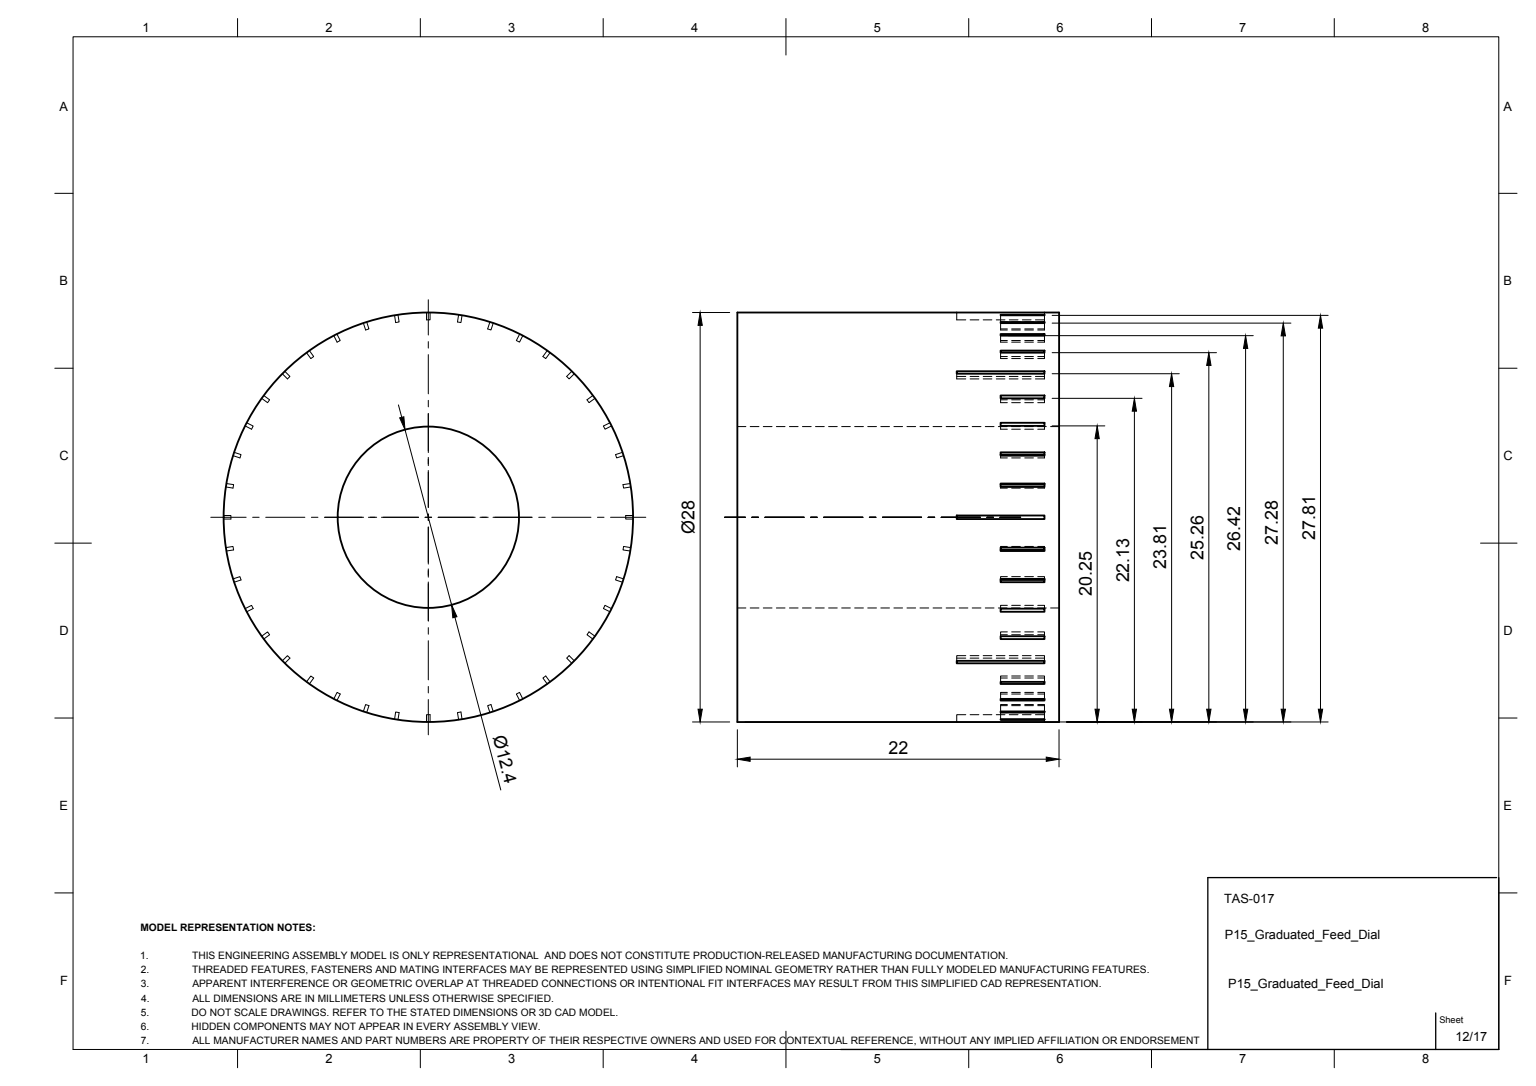
ISO-10303-21;
HEADER;
/* Generated by software containing ST-Developer
 * from STEP Tools, Inc. (www.steptools.com) 
 */

FILE_DESCRIPTION(
/* description */ ('STEP AP203'),
/* implementation_level */ '2;1');

FILE_NAME(
/* name */ 'P15_Graduated_Feed_Dial.step',
/* time_stamp */ '2026-11-15T15:04:01-08:00',
/* author */ (''),
/* organization */ (''),
/* preprocessor_version */ 'ST-DEVELOPER v20.2',
/* originating_system */ 'Autodesk Translation Framework v15.17.0.0',
/* authorisation */ '');

FILE_SCHEMA (('AUTOMOTIVE_DESIGN { 1 0 10303 214 3 1 1 }'));
ENDSEC;

DATA;
#10=MECHANICAL_DESIGN_GEOMETRIC_PRESENTATION_REPRESENTATION('',(#298),#16598);
#220=SHAPE_REPRESENTATION_RELATIONSHIP('SRR','None',#16714,#244);
#244=ADVANCED_BREP_SHAPE_REPRESENTATION('',(#268),#16590);
#268=MANIFOLD_SOLID_BREP('Body1',#9803);
#298=STYLED_ITEM('',(#16834),#268);
#374=FACE_BOUND('',#1807,.T.);
#375=FACE_BOUND('',#1808,.T.);
#376=FACE_BOUND('',#1809,.T.);
#377=FACE_BOUND('',#1810,.T.);
#378=FACE_BOUND('',#1811,.T.);
#379=FACE_BOUND('',#1812,.T.);
#380=FACE_BOUND('',#1813,.T.);
#381=FACE_BOUND('',#1814,.T.);
#382=FACE_BOUND('',#1815,.T.);
#383=FACE_BOUND('',#1816,.T.);
#384=FACE_BOUND('',#1817,.T.);
#385=FACE_BOUND('',#1818,.T.);
#386=FACE_BOUND('',#1819,.T.);
#387=FACE_BOUND('',#1820,.T.);
#388=FACE_BOUND('',#1821,.T.);
#389=FACE_BOUND('',#1822,.T.);
#390=FACE_BOUND('',#1823,.T.);
#391=FACE_BOUND('',#1824,.T.);
#392=FACE_BOUND('',#1825,.T.);
#393=FACE_BOUND('',#1826,.T.);
#394=FACE_BOUND('',#1827,.T.);
#395=FACE_BOUND('',#1828,.T.);
#396=FACE_BOUND('',#1829,.T.);
#397=FACE_BOUND('',#1830,.T.);
#398=FACE_BOUND('',#1831,.T.);
#399=FACE_BOUND('',#1832,.T.);
#400=FACE_BOUND('',#1833,.T.);
#401=FACE_BOUND('',#1834,.T.);
#402=FACE_BOUND('',#1835,.T.);
#403=FACE_BOUND('',#1836,.T.);
#404=FACE_BOUND('',#1837,.T.);
#405=FACE_BOUND('',#1838,.T.);
#406=FACE_BOUND('',#1839,.T.);
#407=FACE_BOUND('',#1840,.T.);
#408=FACE_BOUND('',#1841,.T.);
#409=FACE_BOUND('',#1842,.T.);
#410=FACE_BOUND('',#1843,.T.);
#411=FACE_BOUND('',#1844,.T.);
#412=FACE_BOUND('',#1845,.T.);
#413=FACE_BOUND('',#1847,.T.);
#414=FACE_BOUND('',#1849,.T.);
#651=PLANE('',#10576);
#652=PLANE('',#10577);
#653=PLANE('',#10578);
#654=PLANE('',#10579);
#655=PLANE('',#10580);
#656=PLANE('',#10581);
#657=PLANE('',#10582);
#658=PLANE('',#10583);
#659=PLANE('',#10584);
#660=PLANE('',#10585);
#661=PLANE('',#10586);
#662=PLANE('',#10587);
#663=PLANE('',#10588);
#664=PLANE('',#10589);
#665=PLANE('',#10590);
#666=PLANE('',#10591);
#667=PLANE('',#10592);
#668=PLANE('',#10593);
#669=PLANE('',#10594);
#670=PLANE('',#10595);
#671=PLANE('',#10596);
#672=PLANE('',#10597);
#673=PLANE('',#10598);
#674=PLANE('',#10599);
#675=PLANE('',#10600);
#676=PLANE('',#10601);
#677=PLANE('',#10602);
#678=PLANE('',#10603);
#679=PLANE('',#10604);
#680=PLANE('',#10605);
#681=PLANE('',#10606);
#682=PLANE('',#10607);
#683=PLANE('',#10608);
#684=PLANE('',#10609);
#685=PLANE('',#10610);
#686=PLANE('',#10611);
#687=PLANE('',#10612);
#688=PLANE('',#10613);
#689=PLANE('',#10614);
#690=PLANE('',#10615);
#691=PLANE('',#10616);
#692=PLANE('',#10617);
#693=PLANE('',#10618);
#694=PLANE('',#10619);
#695=PLANE('',#10620);
#696=PLANE('',#10621);
#697=PLANE('',#10622);
#698=PLANE('',#10623);
#699=PLANE('',#10624);
#700=PLANE('',#10625);
#701=PLANE('',#10626);
#702=PLANE('',#10627);
#703=PLANE('',#10628);
#704=PLANE('',#10629);
#705=PLANE('',#10630);
#706=PLANE('',#10631);
#707=PLANE('',#10632);
#708=PLANE('',#10633);
#709=PLANE('',#10634);
#710=PLANE('',#10635);
#711=PLANE('',#10636);
#712=PLANE('',#10637);
#713=PLANE('',#10638);
#714=PLANE('',#10639);
#715=PLANE('',#10640);
#716=PLANE('',#10641);
#717=PLANE('',#10642);
#718=PLANE('',#10643);
#719=PLANE('',#10644);
#720=PLANE('',#10645);
#721=PLANE('',#10646);
#722=PLANE('',#10647);
#723=PLANE('',#10648);
#724=PLANE('',#10649);
#725=PLANE('',#10650);
#726=PLANE('',#10651);
#727=PLANE('',#10652);
#728=PLANE('',#10653);
#729=PLANE('',#10654);
#730=PLANE('',#10655);
#731=PLANE('',#10656);
#732=PLANE('',#10657);
#733=PLANE('',#10658);
#734=PLANE('',#10659);
#735=PLANE('',#10660);
#736=PLANE('',#10661);
#737=PLANE('',#10662);
#738=PLANE('',#10663);
#739=PLANE('',#10664);
#740=PLANE('',#10665);
#741=PLANE('',#10666);
#742=PLANE('',#10667);
#743=PLANE('',#10668);
#744=PLANE('',#10669);
#745=PLANE('',#10670);
#746=PLANE('',#10671);
#747=PLANE('',#10672);
#748=PLANE('',#10673);
#749=PLANE('',#10674);
#750=PLANE('',#10675);
#751=PLANE('',#10676);
#752=PLANE('',#10677);
#753=PLANE('',#10678);
#754=PLANE('',#10679);
#755=PLANE('',#10680);
#756=PLANE('',#10681);
#757=PLANE('',#10682);
#758=PLANE('',#10683);
#759=PLANE('',#10684);
#760=PLANE('',#10685);
#761=PLANE('',#10686);
#762=PLANE('',#10687);
#763=PLANE('',#10688);
#764=PLANE('',#10689);
#765=PLANE('',#10690);
#766=PLANE('',#10691);
#767=PLANE('',#10692);
#768=PLANE('',#10693);
#769=PLANE('',#10694);
#770=PLANE('',#10695);
#771=PLANE('',#10696);
#772=PLANE('',#10697);
#773=PLANE('',#10698);
#774=PLANE('',#10699);
#775=PLANE('',#10700);
#776=PLANE('',#10701);
#777=PLANE('',#10702);
#778=PLANE('',#10703);
#779=PLANE('',#10704);
#780=PLANE('',#10705);
#781=PLANE('',#10706);
#782=PLANE('',#10707);
#783=PLANE('',#10708);
#784=PLANE('',#10709);
#785=PLANE('',#10710);
#786=PLANE('',#10711);
#787=PLANE('',#10712);
#788=PLANE('',#10713);
#789=PLANE('',#10714);
#790=PLANE('',#10715);
#791=PLANE('',#10716);
#792=PLANE('',#10717);
#793=PLANE('',#10718);
#794=PLANE('',#10719);
#795=PLANE('',#10720);
#796=PLANE('',#10721);
#797=PLANE('',#10722);
#798=PLANE('',#10723);
#799=PLANE('',#10724);
#800=PLANE('',#10725);
#801=PLANE('',#10726);
#802=PLANE('',#10727);
#803=PLANE('',#10728);
#804=PLANE('',#10729);
#805=PLANE('',#10730);
#806=PLANE('',#10731);
#807=PLANE('',#10732);
#808=PLANE('',#10733);
#809=PLANE('',#10734);
#810=PLANE('',#10735);
#811=PLANE('',#10736);
#812=PLANE('',#10737);
#813=PLANE('',#10738);
#814=PLANE('',#10739);
#815=PLANE('',#10740);
#816=PLANE('',#10741);
#817=PLANE('',#10742);
#818=PLANE('',#10743);
#819=PLANE('',#10744);
#820=PLANE('',#10745);
#821=PLANE('',#10746);
#822=PLANE('',#10747);
#823=PLANE('',#10748);
#824=PLANE('',#10749);
#825=PLANE('',#10750);
#826=PLANE('',#10751);
#827=PLANE('',#10752);
#828=PLANE('',#10753);
#829=PLANE('',#10754);
#830=PLANE('',#10755);
#831=PLANE('',#10756);
#832=PLANE('',#10757);
#833=PLANE('',#10758);
#834=PLANE('',#10759);
#835=PLANE('',#10760);
#836=PLANE('',#10761);
#837=PLANE('',#10762);
#838=PLANE('',#10763);
#839=PLANE('',#10764);
#840=PLANE('',#10765);
#841=PLANE('',#10766);
#842=PLANE('',#10767);
#843=PLANE('',#10768);
#844=PLANE('',#10769);
#845=PLANE('',#10770);
#846=PLANE('',#10771);
#847=PLANE('',#10772);
#848=PLANE('',#10773);
#849=PLANE('',#10774);
#850=PLANE('',#10775);
#851=PLANE('',#10776);
#852=PLANE('',#10777);
#1186=FACE_OUTER_BOUND('',#1805,.T.);
#1187=FACE_OUTER_BOUND('',#1806,.T.);
#1188=FACE_OUTER_BOUND('',#1846,.T.);
#1189=FACE_OUTER_BOUND('',#1848,.T.);
#1190=FACE_OUTER_BOUND('',#1850,.T.);
#1191=FACE_OUTER_BOUND('',#1851,.T.);
#1192=FACE_OUTER_BOUND('',#1852,.T.);
#1193=FACE_OUTER_BOUND('',#1853,.T.);
#1194=FACE_OUTER_BOUND('',#1854,.T.);
#1195=FACE_OUTER_BOUND('',#1855,.T.);
#1196=FACE_OUTER_BOUND('',#1856,.T.);
#1197=FACE_OUTER_BOUND('',#1857,.T.);
#1198=FACE_OUTER_BOUND('',#1858,.T.);
#1199=FACE_OUTER_BOUND('',#1859,.T.);
#1200=FACE_OUTER_BOUND('',#1860,.T.);
#1201=FACE_OUTER_BOUND('',#1861,.T.);
#1202=FACE_OUTER_BOUND('',#1862,.T.);
#1203=FACE_OUTER_BOUND('',#1863,.T.);
#1204=FACE_OUTER_BOUND('',#1864,.T.);
#1205=FACE_OUTER_BOUND('',#1865,.T.);
#1206=FACE_OUTER_BOUND('',#1866,.T.);
#1207=FACE_OUTER_BOUND('',#1867,.T.);
#1208=FACE_OUTER_BOUND('',#1868,.T.);
#1209=FACE_OUTER_BOUND('',#1869,.T.);
#1210=FACE_OUTER_BOUND('',#1870,.T.);
#1211=FACE_OUTER_BOUND('',#1871,.T.);
#1212=FACE_OUTER_BOUND('',#1872,.T.);
#1213=FACE_OUTER_BOUND('',#1873,.T.);
#1214=FACE_OUTER_BOUND('',#1874,.T.);
#1215=FACE_OUTER_BOUND('',#1875,.T.);
#1216=FACE_OUTER_BOUND('',#1876,.T.);
#1217=FACE_OUTER_BOUND('',#1877,.T.);
#1218=FACE_OUTER_BOUND('',#1878,.T.);
#1219=FACE_OUTER_BOUND('',#1879,.T.);
#1220=FACE_OUTER_BOUND('',#1880,.T.);
#1221=FACE_OUTER_BOUND('',#1881,.T.);
#1222=FACE_OUTER_BOUND('',#1882,.T.);
#1223=FACE_OUTER_BOUND('',#1883,.T.);
#1224=FACE_OUTER_BOUND('',#1884,.T.);
#1225=FACE_OUTER_BOUND('',#1885,.T.);
#1226=FACE_OUTER_BOUND('',#1886,.T.);
#1227=FACE_OUTER_BOUND('',#1887,.T.);
#1228=FACE_OUTER_BOUND('',#1888,.T.);
#1229=FACE_OUTER_BOUND('',#1889,.T.);
#1230=FACE_OUTER_BOUND('',#1890,.T.);
#1231=FACE_OUTER_BOUND('',#1891,.T.);
#1232=FACE_OUTER_BOUND('',#1892,.T.);
#1233=FACE_OUTER_BOUND('',#1893,.T.);
#1234=FACE_OUTER_BOUND('',#1894,.T.);
#1235=FACE_OUTER_BOUND('',#1895,.T.);
#1236=FACE_OUTER_BOUND('',#1896,.T.);
#1237=FACE_OUTER_BOUND('',#1897,.T.);
#1238=FACE_OUTER_BOUND('',#1898,.T.);
#1239=FACE_OUTER_BOUND('',#1899,.T.);
#1240=FACE_OUTER_BOUND('',#1900,.T.);
#1241=FACE_OUTER_BOUND('',#1901,.T.);
#1242=FACE_OUTER_BOUND('',#1902,.T.);
#1243=FACE_OUTER_BOUND('',#1903,.T.);
#1244=FACE_OUTER_BOUND('',#1904,.T.);
#1245=FACE_OUTER_BOUND('',#1905,.T.);
#1246=FACE_OUTER_BOUND('',#1906,.T.);
#1247=FACE_OUTER_BOUND('',#1907,.T.);
#1248=FACE_OUTER_BOUND('',#1908,.T.);
#1249=FACE_OUTER_BOUND('',#1909,.T.);
#1250=FACE_OUTER_BOUND('',#1910,.T.);
#1251=FACE_OUTER_BOUND('',#1911,.T.);
#1252=FACE_OUTER_BOUND('',#1912,.T.);
#1253=FACE_OUTER_BOUND('',#1913,.T.);
#1254=FACE_OUTER_BOUND('',#1914,.T.);
#1255=FACE_OUTER_BOUND('',#1915,.T.);
#1256=FACE_OUTER_BOUND('',#1916,.T.);
#1257=FACE_OUTER_BOUND('',#1917,.T.);
#1258=FACE_OUTER_BOUND('',#1918,.T.);
#1259=FACE_OUTER_BOUND('',#1919,.T.);
#1260=FACE_OUTER_BOUND('',#1920,.T.);
#1261=FACE_OUTER_BOUND('',#1921,.T.);
#1262=FACE_OUTER_BOUND('',#1922,.T.);
#1263=FACE_OUTER_BOUND('',#1923,.T.);
#1264=FACE_OUTER_BOUND('',#1924,.T.);
#1265=FACE_OUTER_BOUND('',#1925,.T.);
#1266=FACE_OUTER_BOUND('',#1926,.T.);
#1267=FACE_OUTER_BOUND('',#1927,.T.);
#1268=FACE_OUTER_BOUND('',#1928,.T.);
#1269=FACE_OUTER_BOUND('',#1929,.T.);
#1270=FACE_OUTER_BOUND('',#1930,.T.);
#1271=FACE_OUTER_BOUND('',#1931,.T.);
#1272=FACE_OUTER_BOUND('',#1932,.T.);
#1273=FACE_OUTER_BOUND('',#1933,.T.);
#1274=FACE_OUTER_BOUND('',#1934,.T.);
#1275=FACE_OUTER_BOUND('',#1935,.T.);
#1276=FACE_OUTER_BOUND('',#1936,.T.);
#1277=FACE_OUTER_BOUND('',#1937,.T.);
#1278=FACE_OUTER_BOUND('',#1938,.T.);
#1279=FACE_OUTER_BOUND('',#1939,.T.);
#1280=FACE_OUTER_BOUND('',#1940,.T.);
#1281=FACE_OUTER_BOUND('',#1941,.T.);
#1282=FACE_OUTER_BOUND('',#1942,.T.);
#1283=FACE_OUTER_BOUND('',#1943,.T.);
#1284=FACE_OUTER_BOUND('',#1944,.T.);
#1285=FACE_OUTER_BOUND('',#1945,.T.);
#1286=FACE_OUTER_BOUND('',#1946,.T.);
#1287=FACE_OUTER_BOUND('',#1947,.T.);
#1288=FACE_OUTER_BOUND('',#1948,.T.);
#1289=FACE_OUTER_BOUND('',#1949,.T.);
#1290=FACE_OUTER_BOUND('',#1950,.T.);
#1291=FACE_OUTER_BOUND('',#1951,.T.);
#1292=FACE_OUTER_BOUND('',#1952,.T.);
#1293=FACE_OUTER_BOUND('',#1953,.T.);
#1294=FACE_OUTER_BOUND('',#1954,.T.);
#1295=FACE_OUTER_BOUND('',#1955,.T.);
#1296=FACE_OUTER_BOUND('',#1956,.T.);
#1297=FACE_OUTER_BOUND('',#1957,.T.);
#1298=FACE_OUTER_BOUND('',#1958,.T.);
#1299=FACE_OUTER_BOUND('',#1959,.T.);
#1300=FACE_OUTER_BOUND('',#1960,.T.);
#1301=FACE_OUTER_BOUND('',#1961,.T.);
#1302=FACE_OUTER_BOUND('',#1962,.T.);
#1303=FACE_OUTER_BOUND('',#1963,.T.);
#1304=FACE_OUTER_BOUND('',#1964,.T.);
#1305=FACE_OUTER_BOUND('',#1965,.T.);
#1306=FACE_OUTER_BOUND('',#1966,.T.);
#1307=FACE_OUTER_BOUND('',#1967,.T.);
#1308=FACE_OUTER_BOUND('',#1968,.T.);
#1309=FACE_OUTER_BOUND('',#1969,.T.);
#1310=FACE_OUTER_BOUND('',#1970,.T.);
#1311=FACE_OUTER_BOUND('',#1971,.T.);
#1312=FACE_OUTER_BOUND('',#1972,.T.);
#1313=FACE_OUTER_BOUND('',#1973,.T.);
#1314=FACE_OUTER_BOUND('',#1974,.T.);
#1315=FACE_OUTER_BOUND('',#1975,.T.);
#1316=FACE_OUTER_BOUND('',#1976,.T.);
#1317=FACE_OUTER_BOUND('',#1977,.T.);
#1318=FACE_OUTER_BOUND('',#1978,.T.);
#1319=FACE_OUTER_BOUND('',#1979,.T.);
#1320=FACE_OUTER_BOUND('',#1980,.T.);
#1321=FACE_OUTER_BOUND('',#1981,.T.);
#1322=FACE_OUTER_BOUND('',#1982,.T.);
#1323=FACE_OUTER_BOUND('',#1983,.T.);
#1324=FACE_OUTER_BOUND('',#1984,.T.);
#1325=FACE_OUTER_BOUND('',#1985,.T.);
#1326=FACE_OUTER_BOUND('',#1986,.T.);
#1327=FACE_OUTER_BOUND('',#1987,.T.);
#1328=FACE_OUTER_BOUND('',#1988,.T.);
#1329=FACE_OUTER_BOUND('',#1989,.T.);
#1330=FACE_OUTER_BOUND('',#1990,.T.);
#1331=FACE_OUTER_BOUND('',#1991,.T.);
#1332=FACE_OUTER_BOUND('',#1992,.T.);
#1333=FACE_OUTER_BOUND('',#1993,.T.);
#1334=FACE_OUTER_BOUND('',#1994,.T.);
#1335=FACE_OUTER_BOUND('',#1995,.T.);
#1336=FACE_OUTER_BOUND('',#1996,.T.);
#1337=FACE_OUTER_BOUND('',#1997,.T.);
#1338=FACE_OUTER_BOUND('',#1998,.T.);
#1339=FACE_OUTER_BOUND('',#1999,.T.);
#1340=FACE_OUTER_BOUND('',#2000,.T.);
#1341=FACE_OUTER_BOUND('',#2001,.T.);
#1342=FACE_OUTER_BOUND('',#2002,.T.);
#1343=FACE_OUTER_BOUND('',#2003,.T.);
#1344=FACE_OUTER_BOUND('',#2004,.T.);
#1345=FACE_OUTER_BOUND('',#2005,.T.);
#1346=FACE_OUTER_BOUND('',#2006,.T.);
#1347=FACE_OUTER_BOUND('',#2007,.T.);
#1348=FACE_OUTER_BOUND('',#2008,.T.);
#1349=FACE_OUTER_BOUND('',#2009,.T.);
#1350=FACE_OUTER_BOUND('',#2010,.T.);
#1351=FACE_OUTER_BOUND('',#2011,.T.);
#1352=FACE_OUTER_BOUND('',#2012,.T.);
#1353=FACE_OUTER_BOUND('',#2013,.T.);
#1354=FACE_OUTER_BOUND('',#2014,.T.);
#1355=FACE_OUTER_BOUND('',#2015,.T.);
#1356=FACE_OUTER_BOUND('',#2016,.T.);
#1357=FACE_OUTER_BOUND('',#2017,.T.);
#1358=FACE_OUTER_BOUND('',#2018,.T.);
#1359=FACE_OUTER_BOUND('',#2019,.T.);
#1360=FACE_OUTER_BOUND('',#2020,.T.);
#1361=FACE_OUTER_BOUND('',#2021,.T.);
#1362=FACE_OUTER_BOUND('',#2022,.T.);
#1363=FACE_OUTER_BOUND('',#2023,.T.);
#1364=FACE_OUTER_BOUND('',#2024,.T.);
#1365=FACE_OUTER_BOUND('',#2025,.T.);
#1366=FACE_OUTER_BOUND('',#2026,.T.);
#1367=FACE_OUTER_BOUND('',#2027,.T.);
#1368=FACE_OUTER_BOUND('',#2028,.T.);
#1369=FACE_OUTER_BOUND('',#2029,.T.);
#1370=FACE_OUTER_BOUND('',#2030,.T.);
#1371=FACE_OUTER_BOUND('',#2031,.T.);
#1372=FACE_OUTER_BOUND('',#2032,.T.);
#1373=FACE_OUTER_BOUND('',#2033,.T.);
#1374=FACE_OUTER_BOUND('',#2034,.T.);
#1375=FACE_OUTER_BOUND('',#2035,.T.);
#1376=FACE_OUTER_BOUND('',#2036,.T.);
#1377=FACE_OUTER_BOUND('',#2037,.T.);
#1378=FACE_OUTER_BOUND('',#2038,.T.);
#1379=FACE_OUTER_BOUND('',#2039,.T.);
#1380=FACE_OUTER_BOUND('',#2040,.T.);
#1381=FACE_OUTER_BOUND('',#2041,.T.);
#1382=FACE_OUTER_BOUND('',#2042,.T.);
#1383=FACE_OUTER_BOUND('',#2043,.T.);
#1384=FACE_OUTER_BOUND('',#2044,.T.);
#1385=FACE_OUTER_BOUND('',#2045,.T.);
#1386=FACE_OUTER_BOUND('',#2046,.T.);
#1387=FACE_OUTER_BOUND('',#2047,.T.);
#1388=FACE_OUTER_BOUND('',#2048,.T.);
#1389=FACE_OUTER_BOUND('',#2049,.T.);
#1805=EDGE_LOOP('',(#7881,#7882,#7883,#7884));
#1806=EDGE_LOOP('',(#7885,#7886,#7887,#7888,#7889,#7890,#7891,#7892,#7893,
#7894,#7895,#7896));
#1807=EDGE_LOOP('',(#7897,#7898,#7899,#7900));
#1808=EDGE_LOOP('',(#7901,#7902,#7903,#7904));
#1809=EDGE_LOOP('',(#7905,#7906,#7907,#7908));
#1810=EDGE_LOOP('',(#7909,#7910,#7911,#7912));
#1811=EDGE_LOOP('',(#7913,#7914,#7915,#7916));
#1812=EDGE_LOOP('',(#7917,#7918,#7919,#7920));
#1813=EDGE_LOOP('',(#7921,#7922,#7923,#7924));
#1814=EDGE_LOOP('',(#7925,#7926,#7927,#7928));
#1815=EDGE_LOOP('',(#7929,#7930,#7931,#7932));
#1816=EDGE_LOOP('',(#7933,#7934,#7935,#7936));
#1817=EDGE_LOOP('',(#7937,#7938,#7939,#7940));
#1818=EDGE_LOOP('',(#7941,#7942,#7943,#7944));
#1819=EDGE_LOOP('',(#7945,#7946,#7947,#7948));
#1820=EDGE_LOOP('',(#7949,#7950,#7951,#7952));
#1821=EDGE_LOOP('',(#7953,#7954,#7955,#7956));
#1822=EDGE_LOOP('',(#7957,#7958,#7959,#7960));
#1823=EDGE_LOOP('',(#7961,#7962,#7963,#7964));
#1824=EDGE_LOOP('',(#7965,#7966,#7967,#7968));
#1825=EDGE_LOOP('',(#7969,#7970,#7971,#7972));
#1826=EDGE_LOOP('',(#7973,#7974,#7975,#7976));
#1827=EDGE_LOOP('',(#7977,#7978,#7979,#7980));
#1828=EDGE_LOOP('',(#7981,#7982,#7983,#7984));
#1829=EDGE_LOOP('',(#7985,#7986,#7987,#7988));
#1830=EDGE_LOOP('',(#7989,#7990,#7991,#7992));
#1831=EDGE_LOOP('',(#7993,#7994,#7995,#7996));
#1832=EDGE_LOOP('',(#7997,#7998,#7999,#8000));
#1833=EDGE_LOOP('',(#8001,#8002,#8003,#8004));
#1834=EDGE_LOOP('',(#8005,#8006,#8007,#8008));
#1835=EDGE_LOOP('',(#8009,#8010,#8011,#8012));
#1836=EDGE_LOOP('',(#8013,#8014,#8015,#8016));
#1837=EDGE_LOOP('',(#8017,#8018,#8019,#8020));
#1838=EDGE_LOOP('',(#8021,#8022,#8023,#8024));
#1839=EDGE_LOOP('',(#8025,#8026,#8027,#8028));
#1840=EDGE_LOOP('',(#8029,#8030,#8031,#8032));
#1841=EDGE_LOOP('',(#8033,#8034,#8035,#8036));
#1842=EDGE_LOOP('',(#8037,#8038,#8039,#8040));
#1843=EDGE_LOOP('',(#8041,#8042,#8043,#8044));
#1844=EDGE_LOOP('',(#8045,#8046,#8047,#8048));
#1845=EDGE_LOOP('',(#8049,#8050,#8051,#8052));
#1846=EDGE_LOOP('',(#8053));
#1847=EDGE_LOOP('',(#8054));
#1848=EDGE_LOOP('',(#8055));
#1849=EDGE_LOOP('',(#8056));
#1850=EDGE_LOOP('',(#8057,#8058,#8059,#8060));
#1851=EDGE_LOOP('',(#8061,#8062,#8063,#8064));
#1852=EDGE_LOOP('',(#8065,#8066,#8067,#8068));
#1853=EDGE_LOOP('',(#8069,#8070,#8071,#8072));
#1854=EDGE_LOOP('',(#8073,#8074,#8075,#8076));
#1855=EDGE_LOOP('',(#8077,#8078,#8079,#8080));
#1856=EDGE_LOOP('',(#8081,#8082,#8083,#8084));
#1857=EDGE_LOOP('',(#8085,#8086,#8087,#8088));
#1858=EDGE_LOOP('',(#8089,#8090,#8091,#8092));
#1859=EDGE_LOOP('',(#8093,#8094,#8095,#8096));
#1860=EDGE_LOOP('',(#8097,#8098,#8099,#8100));
#1861=EDGE_LOOP('',(#8101,#8102,#8103,#8104));
#1862=EDGE_LOOP('',(#8105,#8106,#8107,#8108));
#1863=EDGE_LOOP('',(#8109,#8110,#8111,#8112));
#1864=EDGE_LOOP('',(#8113,#8114,#8115,#8116));
#1865=EDGE_LOOP('',(#8117,#8118,#8119,#8120));
#1866=EDGE_LOOP('',(#8121,#8122,#8123,#8124));
#1867=EDGE_LOOP('',(#8125,#8126,#8127,#8128));
#1868=EDGE_LOOP('',(#8129,#8130,#8131,#8132));
#1869=EDGE_LOOP('',(#8133,#8134,#8135,#8136));
#1870=EDGE_LOOP('',(#8137,#8138,#8139,#8140));
#1871=EDGE_LOOP('',(#8141,#8142,#8143,#8144));
#1872=EDGE_LOOP('',(#8145,#8146,#8147,#8148));
#1873=EDGE_LOOP('',(#8149,#8150,#8151,#8152));
#1874=EDGE_LOOP('',(#8153,#8154,#8155,#8156));
#1875=EDGE_LOOP('',(#8157,#8158,#8159,#8160));
#1876=EDGE_LOOP('',(#8161,#8162,#8163,#8164));
#1877=EDGE_LOOP('',(#8165,#8166,#8167,#8168));
#1878=EDGE_LOOP('',(#8169,#8170,#8171,#8172));
#1879=EDGE_LOOP('',(#8173,#8174,#8175,#8176));
#1880=EDGE_LOOP('',(#8177,#8178,#8179,#8180));
#1881=EDGE_LOOP('',(#8181,#8182,#8183,#8184));
#1882=EDGE_LOOP('',(#8185,#8186,#8187,#8188));
#1883=EDGE_LOOP('',(#8189,#8190,#8191,#8192));
#1884=EDGE_LOOP('',(#8193,#8194,#8195,#8196));
#1885=EDGE_LOOP('',(#8197,#8198,#8199,#8200));
#1886=EDGE_LOOP('',(#8201,#8202,#8203,#8204));
#1887=EDGE_LOOP('',(#8205,#8206,#8207,#8208,#8209));
#1888=EDGE_LOOP('',(#8210,#8211,#8212,#8213,#8214));
#1889=EDGE_LOOP('',(#8215,#8216,#8217,#8218));
#1890=EDGE_LOOP('',(#8219,#8220,#8221,#8222));
#1891=EDGE_LOOP('',(#8223,#8224,#8225,#8226));
#1892=EDGE_LOOP('',(#8227,#8228,#8229,#8230));
#1893=EDGE_LOOP('',(#8231,#8232,#8233,#8234));
#1894=EDGE_LOOP('',(#8235,#8236,#8237,#8238));
#1895=EDGE_LOOP('',(#8239,#8240,#8241,#8242));
#1896=EDGE_LOOP('',(#8243,#8244,#8245,#8246));
#1897=EDGE_LOOP('',(#8247,#8248,#8249,#8250));
#1898=EDGE_LOOP('',(#8251,#8252,#8253,#8254));
#1899=EDGE_LOOP('',(#8255,#8256,#8257,#8258));
#1900=EDGE_LOOP('',(#8259,#8260,#8261,#8262));
#1901=EDGE_LOOP('',(#8263,#8264,#8265,#8266));
#1902=EDGE_LOOP('',(#8267,#8268,#8269,#8270));
#1903=EDGE_LOOP('',(#8271,#8272,#8273,#8274));
#1904=EDGE_LOOP('',(#8275,#8276,#8277,#8278));
#1905=EDGE_LOOP('',(#8279,#8280,#8281,#8282));
#1906=EDGE_LOOP('',(#8283,#8284,#8285,#8286));
#1907=EDGE_LOOP('',(#8287,#8288,#8289,#8290));
#1908=EDGE_LOOP('',(#8291,#8292,#8293,#8294));
#1909=EDGE_LOOP('',(#8295,#8296,#8297,#8298));
#1910=EDGE_LOOP('',(#8299,#8300,#8301,#8302));
#1911=EDGE_LOOP('',(#8303,#8304,#8305,#8306));
#1912=EDGE_LOOP('',(#8307,#8308,#8309,#8310));
#1913=EDGE_LOOP('',(#8311,#8312,#8313,#8314));
#1914=EDGE_LOOP('',(#8315,#8316,#8317,#8318));
#1915=EDGE_LOOP('',(#8319,#8320,#8321,#8322));
#1916=EDGE_LOOP('',(#8323,#8324,#8325,#8326));
#1917=EDGE_LOOP('',(#8327,#8328,#8329,#8330));
#1918=EDGE_LOOP('',(#8331,#8332,#8333,#8334));
#1919=EDGE_LOOP('',(#8335,#8336,#8337,#8338));
#1920=EDGE_LOOP('',(#8339,#8340,#8341,#8342));
#1921=EDGE_LOOP('',(#8343,#8344,#8345,#8346));
#1922=EDGE_LOOP('',(#8347,#8348,#8349,#8350));
#1923=EDGE_LOOP('',(#8351,#8352,#8353,#8354));
#1924=EDGE_LOOP('',(#8355,#8356,#8357,#8358));
#1925=EDGE_LOOP('',(#8359,#8360,#8361,#8362));
#1926=EDGE_LOOP('',(#8363,#8364,#8365,#8366));
#1927=EDGE_LOOP('',(#8367,#8368,#8369,#8370));
#1928=EDGE_LOOP('',(#8371,#8372,#8373,#8374));
#1929=EDGE_LOOP('',(#8375,#8376,#8377,#8378));
#1930=EDGE_LOOP('',(#8379,#8380,#8381,#8382));
#1931=EDGE_LOOP('',(#8383,#8384,#8385,#8386));
#1932=EDGE_LOOP('',(#8387,#8388,#8389,#8390));
#1933=EDGE_LOOP('',(#8391,#8392,#8393,#8394));
#1934=EDGE_LOOP('',(#8395,#8396,#8397,#8398));
#1935=EDGE_LOOP('',(#8399,#8400,#8401,#8402));
#1936=EDGE_LOOP('',(#8403,#8404,#8405,#8406));
#1937=EDGE_LOOP('',(#8407,#8408,#8409,#8410));
#1938=EDGE_LOOP('',(#8411,#8412,#8413,#8414));
#1939=EDGE_LOOP('',(#8415,#8416,#8417,#8418));
#1940=EDGE_LOOP('',(#8419,#8420,#8421,#8422));
#1941=EDGE_LOOP('',(#8423,#8424,#8425,#8426));
#1942=EDGE_LOOP('',(#8427,#8428,#8429,#8430));
#1943=EDGE_LOOP('',(#8431,#8432,#8433,#8434));
#1944=EDGE_LOOP('',(#8435,#8436,#8437,#8438));
#1945=EDGE_LOOP('',(#8439,#8440,#8441,#8442));
#1946=EDGE_LOOP('',(#8443,#8444,#8445,#8446));
#1947=EDGE_LOOP('',(#8447,#8448,#8449,#8450));
#1948=EDGE_LOOP('',(#8451,#8452,#8453,#8454));
#1949=EDGE_LOOP('',(#8455,#8456,#8457,#8458));
#1950=EDGE_LOOP('',(#8459,#8460,#8461,#8462));
#1951=EDGE_LOOP('',(#8463,#8464,#8465,#8466));
#1952=EDGE_LOOP('',(#8467,#8468,#8469,#8470));
#1953=EDGE_LOOP('',(#8471,#8472,#8473,#8474));
#1954=EDGE_LOOP('',(#8475,#8476,#8477,#8478));
#1955=EDGE_LOOP('',(#8479,#8480,#8481,#8482));
#1956=EDGE_LOOP('',(#8483,#8484,#8485,#8486));
#1957=EDGE_LOOP('',(#8487,#8488,#8489,#8490));
#1958=EDGE_LOOP('',(#8491,#8492,#8493,#8494));
#1959=EDGE_LOOP('',(#8495,#8496,#8497,#8498));
#1960=EDGE_LOOP('',(#8499,#8500,#8501,#8502));
#1961=EDGE_LOOP('',(#8503,#8504,#8505,#8506));
#1962=EDGE_LOOP('',(#8507,#8508,#8509,#8510));
#1963=EDGE_LOOP('',(#8511,#8512,#8513,#8514));
#1964=EDGE_LOOP('',(#8515,#8516,#8517,#8518));
#1965=EDGE_LOOP('',(#8519,#8520,#8521,#8522));
#1966=EDGE_LOOP('',(#8523,#8524,#8525,#8526));
#1967=EDGE_LOOP('',(#8527,#8528,#8529,#8530));
#1968=EDGE_LOOP('',(#8531,#8532,#8533,#8534));
#1969=EDGE_LOOP('',(#8535,#8536,#8537,#8538));
#1970=EDGE_LOOP('',(#8539,#8540,#8541,#8542));
#1971=EDGE_LOOP('',(#8543,#8544,#8545,#8546));
#1972=EDGE_LOOP('',(#8547,#8548,#8549,#8550));
#1973=EDGE_LOOP('',(#8551,#8552,#8553,#8554));
#1974=EDGE_LOOP('',(#8555,#8556,#8557,#8558));
#1975=EDGE_LOOP('',(#8559,#8560,#8561,#8562));
#1976=EDGE_LOOP('',(#8563,#8564,#8565,#8566));
#1977=EDGE_LOOP('',(#8567,#8568,#8569,#8570));
#1978=EDGE_LOOP('',(#8571,#8572,#8573,#8574));
#1979=EDGE_LOOP('',(#8575,#8576,#8577,#8578));
#1980=EDGE_LOOP('',(#8579,#8580,#8581,#8582));
#1981=EDGE_LOOP('',(#8583,#8584,#8585,#8586));
#1982=EDGE_LOOP('',(#8587,#8588,#8589,#8590));
#1983=EDGE_LOOP('',(#8591,#8592,#8593,#8594));
#1984=EDGE_LOOP('',(#8595,#8596,#8597,#8598));
#1985=EDGE_LOOP('',(#8599,#8600,#8601,#8602));
#1986=EDGE_LOOP('',(#8603,#8604,#8605,#8606));
#1987=EDGE_LOOP('',(#8607,#8608,#8609,#8610));
#1988=EDGE_LOOP('',(#8611,#8612,#8613,#8614));
#1989=EDGE_LOOP('',(#8615,#8616,#8617,#8618));
#1990=EDGE_LOOP('',(#8619,#8620,#8621,#8622));
#1991=EDGE_LOOP('',(#8623,#8624,#8625,#8626));
#1992=EDGE_LOOP('',(#8627,#8628,#8629,#8630));
#1993=EDGE_LOOP('',(#8631,#8632,#8633,#8634));
#1994=EDGE_LOOP('',(#8635,#8636,#8637,#8638));
#1995=EDGE_LOOP('',(#8639,#8640,#8641,#8642));
#1996=EDGE_LOOP('',(#8643,#8644,#8645,#8646));
#1997=EDGE_LOOP('',(#8647,#8648,#8649,#8650));
#1998=EDGE_LOOP('',(#8651,#8652,#8653,#8654));
#1999=EDGE_LOOP('',(#8655,#8656,#8657,#8658));
#2000=EDGE_LOOP('',(#8659,#8660,#8661,#8662));
#2001=EDGE_LOOP('',(#8663,#8664,#8665,#8666));
#2002=EDGE_LOOP('',(#8667,#8668,#8669,#8670));
#2003=EDGE_LOOP('',(#8671,#8672,#8673,#8674));
#2004=EDGE_LOOP('',(#8675,#8676,#8677,#8678));
#2005=EDGE_LOOP('',(#8679,#8680,#8681,#8682));
#2006=EDGE_LOOP('',(#8683,#8684,#8685,#8686));
#2007=EDGE_LOOP('',(#8687,#8688,#8689,#8690));
#2008=EDGE_LOOP('',(#8691,#8692,#8693,#8694));
#2009=EDGE_LOOP('',(#8695,#8696,#8697,#8698));
#2010=EDGE_LOOP('',(#8699,#8700,#8701,#8702));
#2011=EDGE_LOOP('',(#8703,#8704,#8705,#8706));
#2012=EDGE_LOOP('',(#8707,#8708,#8709,#8710));
#2013=EDGE_LOOP('',(#8711,#8712,#8713,#8714));
#2014=EDGE_LOOP('',(#8715,#8716,#8717,#8718));
#2015=EDGE_LOOP('',(#8719,#8720,#8721,#8722));
#2016=EDGE_LOOP('',(#8723,#8724,#8725,#8726));
#2017=EDGE_LOOP('',(#8727,#8728,#8729,#8730));
#2018=EDGE_LOOP('',(#8731,#8732,#8733,#8734));
#2019=EDGE_LOOP('',(#8735,#8736,#8737,#8738));
#2020=EDGE_LOOP('',(#8739,#8740,#8741,#8742));
#2021=EDGE_LOOP('',(#8743,#8744,#8745,#8746));
#2022=EDGE_LOOP('',(#8747,#8748,#8749,#8750));
#2023=EDGE_LOOP('',(#8751,#8752,#8753,#8754));
#2024=EDGE_LOOP('',(#8755,#8756,#8757,#8758));
#2025=EDGE_LOOP('',(#8759,#8760,#8761,#8762));
#2026=EDGE_LOOP('',(#8763,#8764,#8765,#8766));
#2027=EDGE_LOOP('',(#8767,#8768,#8769,#8770));
#2028=EDGE_LOOP('',(#8771,#8772,#8773,#8774));
#2029=EDGE_LOOP('',(#8775,#8776,#8777,#8778));
#2030=EDGE_LOOP('',(#8779,#8780,#8781,#8782));
#2031=EDGE_LOOP('',(#8783,#8784,#8785,#8786));
#2032=EDGE_LOOP('',(#8787,#8788,#8789,#8790));
#2033=EDGE_LOOP('',(#8791,#8792,#8793,#8794));
#2034=EDGE_LOOP('',(#8795,#8796,#8797,#8798));
#2035=EDGE_LOOP('',(#8799,#8800,#8801,#8802));
#2036=EDGE_LOOP('',(#8803,#8804,#8805,#8806));
#2037=EDGE_LOOP('',(#8807,#8808,#8809,#8810));
#2038=EDGE_LOOP('',(#8811,#8812,#8813,#8814));
#2039=EDGE_LOOP('',(#8815,#8816,#8817,#8818));
#2040=EDGE_LOOP('',(#8819,#8820,#8821,#8822));
#2041=EDGE_LOOP('',(#8823,#8824,#8825,#8826));
#2042=EDGE_LOOP('',(#8827,#8828,#8829,#8830));
#2043=EDGE_LOOP('',(#8831,#8832,#8833,#8834));
#2044=EDGE_LOOP('',(#8835,#8836,#8837,#8838));
#2045=EDGE_LOOP('',(#8839,#8840,#8841,#8842));
#2046=EDGE_LOOP('',(#8843,#8844,#8845,#8846));
#2047=EDGE_LOOP('',(#8847,#8848,#8849,#8850));
#2048=EDGE_LOOP('',(#8851,#8852,#8853,#8854));
#2049=EDGE_LOOP('',(#8855,#8856,#8857,#8858));
#2653=LINE('',#15151,#3701);
#2654=LINE('',#15157,#3702);
#2655=LINE('',#15161,#3703);
#2656=LINE('',#15165,#3704);
#2657=LINE('',#15170,#3705);
#2658=LINE('',#15176,#3706);
#2659=LINE('',#15179,#3707);
#2660=LINE('',#15182,#3708);
#2661=LINE('',#15186,#3709);
#2662=LINE('',#15190,#3710);
#2663=LINE('',#15194,#3711);
#2664=LINE('',#15198,#3712);
#2665=LINE('',#15202,#3713);
#2666=LINE('',#15206,#3714);
#2667=LINE('',#15210,#3715);
#2668=LINE('',#15214,#3716);
#2669=LINE('',#15218,#3717);
#2670=LINE('',#15222,#3718);
#2671=LINE('',#15226,#3719);
#2672=LINE('',#15230,#3720);
#2673=LINE('',#15234,#3721);
#2674=LINE('',#15238,#3722);
#2675=LINE('',#15242,#3723);
#2676=LINE('',#15246,#3724);
#2677=LINE('',#15250,#3725);
#2678=LINE('',#15254,#3726);
#2679=LINE('',#15258,#3727);
#2680=LINE('',#15262,#3728);
#2681=LINE('',#15266,#3729);
#2682=LINE('',#15270,#3730);
#2683=LINE('',#15274,#3731);
#2684=LINE('',#15278,#3732);
#2685=LINE('',#15282,#3733);
#2686=LINE('',#15286,#3734);
#2687=LINE('',#15290,#3735);
#2688=LINE('',#15294,#3736);
#2689=LINE('',#15298,#3737);
#2690=LINE('',#15302,#3738);
#2691=LINE('',#15306,#3739);
#2692=LINE('',#15310,#3740);
#2693=LINE('',#15314,#3741);
#2694=LINE('',#15318,#3742);
#2695=LINE('',#15322,#3743);
#2696=LINE('',#15326,#3744);
#2697=LINE('',#15330,#3745);
#2698=LINE('',#15334,#3746);
#2699=LINE('',#15338,#3747);
#2700=LINE('',#15342,#3748);
#2701=LINE('',#15346,#3749);
#2702=LINE('',#15350,#3750);
#2703=LINE('',#15354,#3751);
#2704=LINE('',#15358,#3752);
#2705=LINE('',#15362,#3753);
#2706=LINE('',#15366,#3754);
#2707=LINE('',#15370,#3755);
#2708=LINE('',#15374,#3756);
#2709=LINE('',#15378,#3757);
#2710=LINE('',#15382,#3758);
#2711=LINE('',#15386,#3759);
#2712=LINE('',#15390,#3760);
#2713=LINE('',#15394,#3761);
#2714=LINE('',#15398,#3762);
#2715=LINE('',#15402,#3763);
#2716=LINE('',#15406,#3764);
#2717=LINE('',#15410,#3765);
#2718=LINE('',#15414,#3766);
#2719=LINE('',#15418,#3767);
#2720=LINE('',#15422,#3768);
#2721=LINE('',#15426,#3769);
#2722=LINE('',#15430,#3770);
#2723=LINE('',#15434,#3771);
#2724=LINE('',#15438,#3772);
#2725=LINE('',#15442,#3773);
#2726=LINE('',#15446,#3774);
#2727=LINE('',#15450,#3775);
#2728=LINE('',#15454,#3776);
#2729=LINE('',#15458,#3777);
#2730=LINE('',#15462,#3778);
#2731=LINE('',#15466,#3779);
#2732=LINE('',#15470,#3780);
#2733=LINE('',#15474,#3781);
#2734=LINE('',#15478,#3782);
#2735=LINE('',#15482,#3783);
#2736=LINE('',#15488,#3784);
#2737=LINE('',#15490,#3785);
#2738=LINE('',#15491,#3786);
#2739=LINE('',#15494,#3787);
#2740=LINE('',#15496,#3788);
#2741=LINE('',#15497,#3789);
#2742=LINE('',#15499,#3790);
#2743=LINE('',#15501,#3791);
#2744=LINE('',#15505,#3792);
#2745=LINE('',#15507,#3793);
#2746=LINE('',#15508,#3794);
#2747=LINE('',#15511,#3795);
#2748=LINE('',#15513,#3796);
#2749=LINE('',#15514,#3797);
#2750=LINE('',#15516,#3798);
#2751=LINE('',#15518,#3799);
#2752=LINE('',#15522,#3800);
#2753=LINE('',#15524,#3801);
#2754=LINE('',#15525,#3802);
#2755=LINE('',#15528,#3803);
#2756=LINE('',#15530,#3804);
#2757=LINE('',#15531,#3805);
#2758=LINE('',#15533,#3806);
#2759=LINE('',#15535,#3807);
#2760=LINE('',#15539,#3808);
#2761=LINE('',#15541,#3809);
#2762=LINE('',#15542,#3810);
#2763=LINE('',#15545,#3811);
#2764=LINE('',#15547,#3812);
#2765=LINE('',#15548,#3813);
#2766=LINE('',#15550,#3814);
#2767=LINE('',#15552,#3815);
#2768=LINE('',#15556,#3816);
#2769=LINE('',#15558,#3817);
#2770=LINE('',#15559,#3818);
#2771=LINE('',#15562,#3819);
#2772=LINE('',#15564,#3820);
#2773=LINE('',#15565,#3821);
#2774=LINE('',#15567,#3822);
#2775=LINE('',#15569,#3823);
#2776=LINE('',#15573,#3824);
#2777=LINE('',#15575,#3825);
#2778=LINE('',#15576,#3826);
#2779=LINE('',#15579,#3827);
#2780=LINE('',#15581,#3828);
#2781=LINE('',#15582,#3829);
#2782=LINE('',#15584,#3830);
#2783=LINE('',#15586,#3831);
#2784=LINE('',#15590,#3832);
#2785=LINE('',#15592,#3833);
#2786=LINE('',#15593,#3834);
#2787=LINE('',#15596,#3835);
#2788=LINE('',#15598,#3836);
#2789=LINE('',#15599,#3837);
#2790=LINE('',#15601,#3838);
#2791=LINE('',#15603,#3839);
#2792=LINE('',#15607,#3840);
#2793=LINE('',#15609,#3841);
#2794=LINE('',#15610,#3842);
#2795=LINE('',#15613,#3843);
#2796=LINE('',#15615,#3844);
#2797=LINE('',#15616,#3845);
#2798=LINE('',#15618,#3846);
#2799=LINE('',#15620,#3847);
#2800=LINE('',#15624,#3848);
#2801=LINE('',#15626,#3849);
#2802=LINE('',#15627,#3850);
#2803=LINE('',#15630,#3851);
#2804=LINE('',#15632,#3852);
#2805=LINE('',#15633,#3853);
#2806=LINE('',#15635,#3854);
#2807=LINE('',#15637,#3855);
#2808=LINE('',#15641,#3856);
#2809=LINE('',#15643,#3857);
#2810=LINE('',#15644,#3858);
#2811=LINE('',#15647,#3859);
#2812=LINE('',#15649,#3860);
#2813=LINE('',#15650,#3861);
#2814=LINE('',#15652,#3862);
#2815=LINE('',#15654,#3863);
#2816=LINE('',#15658,#3864);
#2817=LINE('',#15660,#3865);
#2818=LINE('',#15661,#3866);
#2819=LINE('',#15664,#3867);
#2820=LINE('',#15666,#3868);
#2821=LINE('',#15667,#3869);
#2822=LINE('',#15669,#3870);
#2823=LINE('',#15671,#3871);
#2824=LINE('',#15675,#3872);
#2825=LINE('',#15677,#3873);
#2826=LINE('',#15678,#3874);
#2827=LINE('',#15681,#3875);
#2828=LINE('',#15683,#3876);
#2829=LINE('',#15684,#3877);
#2830=LINE('',#15686,#3878);
#2831=LINE('',#15688,#3879);
#2832=LINE('',#15692,#3880);
#2833=LINE('',#15694,#3881);
#2834=LINE('',#15695,#3882);
#2835=LINE('',#15698,#3883);
#2836=LINE('',#15700,#3884);
#2837=LINE('',#15701,#3885);
#2838=LINE('',#15703,#3886);
#2839=LINE('',#15705,#3887);
#2840=LINE('',#15709,#3888);
#2841=LINE('',#15711,#3889);
#2842=LINE('',#15712,#3890);
#2843=LINE('',#15715,#3891);
#2844=LINE('',#15717,#3892);
#2845=LINE('',#15718,#3893);
#2846=LINE('',#15720,#3894);
#2847=LINE('',#15722,#3895);
#2848=LINE('',#15726,#3896);
#2849=LINE('',#15728,#3897);
#2850=LINE('',#15729,#3898);
#2851=LINE('',#15732,#3899);
#2852=LINE('',#15734,#3900);
#2853=LINE('',#15735,#3901);
#2854=LINE('',#15737,#3902);
#2855=LINE('',#15739,#3903);
#2856=LINE('',#15743,#3904);
#2857=LINE('',#15745,#3905);
#2858=LINE('',#15746,#3906);
#2859=LINE('',#15749,#3907);
#2860=LINE('',#15751,#3908);
#2861=LINE('',#15752,#3909);
#2862=LINE('',#15754,#3910);
#2863=LINE('',#15756,#3911);
#2864=LINE('',#15760,#3912);
#2865=LINE('',#15762,#3913);
#2866=LINE('',#15763,#3914);
#2867=LINE('',#15766,#3915);
#2868=LINE('',#15768,#3916);
#2869=LINE('',#15769,#3917);
#2870=LINE('',#15771,#3918);
#2871=LINE('',#15773,#3919);
#2872=LINE('',#15777,#3920);
#2873=LINE('',#15779,#3921);
#2874=LINE('',#15780,#3922);
#2875=LINE('',#15783,#3923);
#2876=LINE('',#15785,#3924);
#2877=LINE('',#15786,#3925);
#2878=LINE('',#15788,#3926);
#2879=LINE('',#15790,#3927);
#2880=LINE('',#15794,#3928);
#2881=LINE('',#15796,#3929);
#2882=LINE('',#15797,#3930);
#2883=LINE('',#15800,#3931);
#2884=LINE('',#15802,#3932);
#2885=LINE('',#15803,#3933);
#2886=LINE('',#15805,#3934);
#2887=LINE('',#15807,#3935);
#2888=LINE('',#15811,#3936);
#2889=LINE('',#15813,#3937);
#2890=LINE('',#15814,#3938);
#2891=LINE('',#15817,#3939);
#2892=LINE('',#15819,#3940);
#2893=LINE('',#15820,#3941);
#2894=LINE('',#15822,#3942);
#2895=LINE('',#15824,#3943);
#2896=LINE('',#15828,#3944);
#2897=LINE('',#15830,#3945);
#2898=LINE('',#15831,#3946);
#2899=LINE('',#15834,#3947);
#2900=LINE('',#15836,#3948);
#2901=LINE('',#15837,#3949);
#2902=LINE('',#15839,#3950);
#2903=LINE('',#15841,#3951);
#2904=LINE('',#15845,#3952);
#2905=LINE('',#15847,#3953);
#2906=LINE('',#15848,#3954);
#2907=LINE('',#15851,#3955);
#2908=LINE('',#15853,#3956);
#2909=LINE('',#15854,#3957);
#2910=LINE('',#15856,#3958);
#2911=LINE('',#15858,#3959);
#2912=LINE('',#15862,#3960);
#2913=LINE('',#15864,#3961);
#2914=LINE('',#15865,#3962);
#2915=LINE('',#15868,#3963);
#2916=LINE('',#15870,#3964);
#2917=LINE('',#15871,#3965);
#2918=LINE('',#15873,#3966);
#2919=LINE('',#15875,#3967);
#2920=LINE('',#15879,#3968);
#2921=LINE('',#15881,#3969);
#2922=LINE('',#15882,#3970);
#2923=LINE('',#15885,#3971);
#2924=LINE('',#15887,#3972);
#2925=LINE('',#15888,#3973);
#2926=LINE('',#15890,#3974);
#2927=LINE('',#15892,#3975);
#2928=LINE('',#15896,#3976);
#2929=LINE('',#15898,#3977);
#2930=LINE('',#15899,#3978);
#2931=LINE('',#15902,#3979);
#2932=LINE('',#15904,#3980);
#2933=LINE('',#15905,#3981);
#2934=LINE('',#15907,#3982);
#2935=LINE('',#15909,#3983);
#2936=LINE('',#15913,#3984);
#2937=LINE('',#15915,#3985);
#2938=LINE('',#15916,#3986);
#2939=LINE('',#15919,#3987);
#2940=LINE('',#15921,#3988);
#2941=LINE('',#15922,#3989);
#2942=LINE('',#15924,#3990);
#2943=LINE('',#15926,#3991);
#2944=LINE('',#15930,#3992);
#2945=LINE('',#15932,#3993);
#2946=LINE('',#15933,#3994);
#2947=LINE('',#15936,#3995);
#2948=LINE('',#15938,#3996);
#2949=LINE('',#15939,#3997);
#2950=LINE('',#15941,#3998);
#2951=LINE('',#15943,#3999);
#2952=LINE('',#15947,#4000);
#2953=LINE('',#15949,#4001);
#2954=LINE('',#15950,#4002);
#2955=LINE('',#15953,#4003);
#2956=LINE('',#15955,#4004);
#2957=LINE('',#15956,#4005);
#2958=LINE('',#15958,#4006);
#2959=LINE('',#15960,#4007);
#2960=LINE('',#15964,#4008);
#2961=LINE('',#15966,#4009);
#2962=LINE('',#15967,#4010);
#2963=LINE('',#15970,#4011);
#2964=LINE('',#15972,#4012);
#2965=LINE('',#15973,#4013);
#2966=LINE('',#15975,#4014);
#2967=LINE('',#15977,#4015);
#2968=LINE('',#15981,#4016);
#2969=LINE('',#15983,#4017);
#2970=LINE('',#15984,#4018);
#2971=LINE('',#15987,#4019);
#2972=LINE('',#15989,#4020);
#2973=LINE('',#15990,#4021);
#2974=LINE('',#15992,#4022);
#2975=LINE('',#15994,#4023);
#2976=LINE('',#15998,#4024);
#2977=LINE('',#16000,#4025);
#2978=LINE('',#16001,#4026);
#2979=LINE('',#16004,#4027);
#2980=LINE('',#16006,#4028);
#2981=LINE('',#16007,#4029);
#2982=LINE('',#16009,#4030);
#2983=LINE('',#16011,#4031);
#2984=LINE('',#16015,#4032);
#2985=LINE('',#16017,#4033);
#2986=LINE('',#16018,#4034);
#2987=LINE('',#16021,#4035);
#2988=LINE('',#16023,#4036);
#2989=LINE('',#16024,#4037);
#2990=LINE('',#16026,#4038);
#2991=LINE('',#16028,#4039);
#2992=LINE('',#16032,#4040);
#2993=LINE('',#16034,#4041);
#2994=LINE('',#16035,#4042);
#2995=LINE('',#16038,#4043);
#2996=LINE('',#16040,#4044);
#2997=LINE('',#16041,#4045);
#2998=LINE('',#16043,#4046);
#2999=LINE('',#16045,#4047);
#3000=LINE('',#16049,#4048);
#3001=LINE('',#16051,#4049);
#3002=LINE('',#16052,#4050);
#3003=LINE('',#16055,#4051);
#3004=LINE('',#16057,#4052);
#3005=LINE('',#16058,#4053);
#3006=LINE('',#16060,#4054);
#3007=LINE('',#16062,#4055);
#3008=LINE('',#16066,#4056);
#3009=LINE('',#16068,#4057);
#3010=LINE('',#16069,#4058);
#3011=LINE('',#16072,#4059);
#3012=LINE('',#16074,#4060);
#3013=LINE('',#16075,#4061);
#3014=LINE('',#16077,#4062);
#3015=LINE('',#16079,#4063);
#3016=LINE('',#16083,#4064);
#3017=LINE('',#16085,#4065);
#3018=LINE('',#16086,#4066);
#3019=LINE('',#16089,#4067);
#3020=LINE('',#16091,#4068);
#3021=LINE('',#16092,#4069);
#3022=LINE('',#16094,#4070);
#3023=LINE('',#16096,#4071);
#3024=LINE('',#16100,#4072);
#3025=LINE('',#16102,#4073);
#3026=LINE('',#16103,#4074);
#3027=LINE('',#16106,#4075);
#3028=LINE('',#16108,#4076);
#3029=LINE('',#16109,#4077);
#3030=LINE('',#16111,#4078);
#3031=LINE('',#16113,#4079);
#3032=LINE('',#16117,#4080);
#3033=LINE('',#16119,#4081);
#3034=LINE('',#16120,#4082);
#3035=LINE('',#16123,#4083);
#3036=LINE('',#16125,#4084);
#3037=LINE('',#16126,#4085);
#3038=LINE('',#16128,#4086);
#3039=LINE('',#16130,#4087);
#3040=LINE('',#16134,#4088);
#3041=LINE('',#16136,#4089);
#3042=LINE('',#16137,#4090);
#3043=LINE('',#16140,#4091);
#3044=LINE('',#16142,#4092);
#3045=LINE('',#16143,#4093);
#3046=LINE('',#16145,#4094);
#3047=LINE('',#16147,#4095);
#3048=LINE('',#16151,#4096);
#3049=LINE('',#16153,#4097);
#3050=LINE('',#16154,#4098);
#3051=LINE('',#16157,#4099);
#3052=LINE('',#16159,#4100);
#3053=LINE('',#16160,#4101);
#3054=LINE('',#16162,#4102);
#3055=LINE('',#16164,#4103);
#3701=VECTOR('',#12273,6.2);
#3702=VECTOR('',#12280,14.);
#3703=VECTOR('',#12283,1000.);
#3704=VECTOR('',#12286,14.);
#3705=VECTOR('',#12291,1000.);
#3706=VECTOR('',#12296,1000.);
#3707=VECTOR('',#12299,1000.);
#3708=VECTOR('',#12300,1000.);
#3709=VECTOR('',#12303,1000.);
#3710=VECTOR('',#12306,1000.);
#3711=VECTOR('',#12309,1000.);
#3712=VECTOR('',#12312,1000.);
#3713=VECTOR('',#12315,1000.);
#3714=VECTOR('',#12318,1000.);
#3715=VECTOR('',#12321,1000.);
#3716=VECTOR('',#12324,1000.);
#3717=VECTOR('',#12327,1000.);
#3718=VECTOR('',#12330,1000.);
#3719=VECTOR('',#12333,1000.);
#3720=VECTOR('',#12336,1000.);
#3721=VECTOR('',#12339,1000.);
#3722=VECTOR('',#12342,1000.);
#3723=VECTOR('',#12345,1000.);
#3724=VECTOR('',#12348,1000.);
#3725=VECTOR('',#12351,1000.);
#3726=VECTOR('',#12354,1000.);
#3727=VECTOR('',#12357,1000.);
#3728=VECTOR('',#12360,1000.);
#3729=VECTOR('',#12363,1000.);
#3730=VECTOR('',#12366,1000.);
#3731=VECTOR('',#12369,1000.);
#3732=VECTOR('',#12372,1000.);
#3733=VECTOR('',#12375,1000.);
#3734=VECTOR('',#12378,1000.);
#3735=VECTOR('',#12381,1000.);
#3736=VECTOR('',#12384,1000.);
#3737=VECTOR('',#12387,1000.);
#3738=VECTOR('',#12390,1000.);
#3739=VECTOR('',#12393,1000.);
#3740=VECTOR('',#12396,1000.);
#3741=VECTOR('',#12399,1000.);
#3742=VECTOR('',#12402,1000.);
#3743=VECTOR('',#12405,1000.);
#3744=VECTOR('',#12408,1000.);
#3745=VECTOR('',#12411,1000.);
#3746=VECTOR('',#12414,1000.);
#3747=VECTOR('',#12417,1000.);
#3748=VECTOR('',#12420,1000.);
#3749=VECTOR('',#12423,1000.);
#3750=VECTOR('',#12426,1000.);
#3751=VECTOR('',#12429,1000.);
#3752=VECTOR('',#12432,1000.);
#3753=VECTOR('',#12435,1000.);
#3754=VECTOR('',#12438,1000.);
#3755=VECTOR('',#12441,1000.);
#3756=VECTOR('',#12444,1000.);
#3757=VECTOR('',#12447,1000.);
#3758=VECTOR('',#12450,1000.);
#3759=VECTOR('',#12453,1000.);
#3760=VECTOR('',#12456,1000.);
#3761=VECTOR('',#12459,1000.);
#3762=VECTOR('',#12462,1000.);
#3763=VECTOR('',#12465,1000.);
#3764=VECTOR('',#12468,1000.);
#3765=VECTOR('',#12471,1000.);
#3766=VECTOR('',#12474,1000.);
#3767=VECTOR('',#12477,1000.);
#3768=VECTOR('',#12480,1000.);
#3769=VECTOR('',#12483,1000.);
#3770=VECTOR('',#12486,1000.);
#3771=VECTOR('',#12489,1000.);
#3772=VECTOR('',#12492,1000.);
#3773=VECTOR('',#12495,1000.);
#3774=VECTOR('',#12498,1000.);
#3775=VECTOR('',#12501,1000.);
#3776=VECTOR('',#12504,1000.);
#3777=VECTOR('',#12507,1000.);
#3778=VECTOR('',#12510,1000.);
#3779=VECTOR('',#12513,1000.);
#3780=VECTOR('',#12516,1000.);
#3781=VECTOR('',#12519,1000.);
#3782=VECTOR('',#12522,1000.);
#3783=VECTOR('',#12525,1000.);
#3784=VECTOR('',#12534,1000.);
#3785=VECTOR('',#12535,1000.);
#3786=VECTOR('',#12536,1000.);
#3787=VECTOR('',#12539,1000.);
#3788=VECTOR('',#12540,1000.);
#3789=VECTOR('',#12541,1000.);
#3790=VECTOR('',#12544,1000.);
#3791=VECTOR('',#12547,1000.);
#3792=VECTOR('',#12552,1000.);
#3793=VECTOR('',#12553,1000.);
#3794=VECTOR('',#12554,1000.);
#3795=VECTOR('',#12557,1000.);
#3796=VECTOR('',#12558,1000.);
#3797=VECTOR('',#12559,1000.);
#3798=VECTOR('',#12562,1000.);
#3799=VECTOR('',#12565,1000.);
#3800=VECTOR('',#12570,1000.);
#3801=VECTOR('',#12571,1000.);
#3802=VECTOR('',#12572,1000.);
#3803=VECTOR('',#12575,1000.);
#3804=VECTOR('',#12576,1000.);
#3805=VECTOR('',#12577,1000.);
#3806=VECTOR('',#12580,1000.);
#3807=VECTOR('',#12583,1000.);
#3808=VECTOR('',#12588,1000.);
#3809=VECTOR('',#12589,1000.);
#3810=VECTOR('',#12590,1000.);
#3811=VECTOR('',#12593,1000.);
#3812=VECTOR('',#12594,1000.);
#3813=VECTOR('',#12595,1000.);
#3814=VECTOR('',#12598,1000.);
#3815=VECTOR('',#12601,1000.);
#3816=VECTOR('',#12606,1000.);
#3817=VECTOR('',#12607,1000.);
#3818=VECTOR('',#12608,1000.);
#3819=VECTOR('',#12611,1000.);
#3820=VECTOR('',#12612,1000.);
#3821=VECTOR('',#12613,1000.);
#3822=VECTOR('',#12616,1000.);
#3823=VECTOR('',#12619,1000.);
#3824=VECTOR('',#12624,1000.);
#3825=VECTOR('',#12625,1000.);
#3826=VECTOR('',#12626,1000.);
#3827=VECTOR('',#12629,1000.);
#3828=VECTOR('',#12630,1000.);
#3829=VECTOR('',#12631,1000.);
#3830=VECTOR('',#12634,1000.);
#3831=VECTOR('',#12637,1000.);
#3832=VECTOR('',#12642,1000.);
#3833=VECTOR('',#12643,1000.);
#3834=VECTOR('',#12644,1000.);
#3835=VECTOR('',#12647,1000.);
#3836=VECTOR('',#12648,1000.);
#3837=VECTOR('',#12649,1000.);
#3838=VECTOR('',#12652,1000.);
#3839=VECTOR('',#12655,1000.);
#3840=VECTOR('',#12660,1000.);
#3841=VECTOR('',#12661,1000.);
#3842=VECTOR('',#12662,1000.);
#3843=VECTOR('',#12665,1000.);
#3844=VECTOR('',#12666,1000.);
#3845=VECTOR('',#12667,1000.);
#3846=VECTOR('',#12670,1000.);
#3847=VECTOR('',#12673,1000.);
#3848=VECTOR('',#12678,1000.);
#3849=VECTOR('',#12679,1000.);
#3850=VECTOR('',#12680,1000.);
#3851=VECTOR('',#12683,1000.);
#3852=VECTOR('',#12684,1000.);
#3853=VECTOR('',#12685,1000.);
#3854=VECTOR('',#12688,1000.);
#3855=VECTOR('',#12691,1000.);
#3856=VECTOR('',#12696,1000.);
#3857=VECTOR('',#12697,1000.);
#3858=VECTOR('',#12698,1000.);
#3859=VECTOR('',#12701,1000.);
#3860=VECTOR('',#12702,1000.);
#3861=VECTOR('',#12703,1000.);
#3862=VECTOR('',#12706,1000.);
#3863=VECTOR('',#12709,1000.);
#3864=VECTOR('',#12714,1000.);
#3865=VECTOR('',#12715,1000.);
#3866=VECTOR('',#12716,1000.);
#3867=VECTOR('',#12719,1000.);
#3868=VECTOR('',#12720,1000.);
#3869=VECTOR('',#12721,1000.);
#3870=VECTOR('',#12724,1000.);
#3871=VECTOR('',#12727,1000.);
#3872=VECTOR('',#12732,1000.);
#3873=VECTOR('',#12733,1000.);
#3874=VECTOR('',#12734,1000.);
#3875=VECTOR('',#12737,1000.);
#3876=VECTOR('',#12738,1000.);
#3877=VECTOR('',#12739,1000.);
#3878=VECTOR('',#12742,1000.);
#3879=VECTOR('',#12745,1000.);
#3880=VECTOR('',#12750,1000.);
#3881=VECTOR('',#12751,1000.);
#3882=VECTOR('',#12752,1000.);
#3883=VECTOR('',#12755,1000.);
#3884=VECTOR('',#12756,1000.);
#3885=VECTOR('',#12757,1000.);
#3886=VECTOR('',#12760,1000.);
#3887=VECTOR('',#12763,1000.);
#3888=VECTOR('',#12768,1000.);
#3889=VECTOR('',#12769,1000.);
#3890=VECTOR('',#12770,1000.);
#3891=VECTOR('',#12773,1000.);
#3892=VECTOR('',#12774,1000.);
#3893=VECTOR('',#12775,1000.);
#3894=VECTOR('',#12778,1000.);
#3895=VECTOR('',#12781,1000.);
#3896=VECTOR('',#12786,1000.);
#3897=VECTOR('',#12787,1000.);
#3898=VECTOR('',#12788,1000.);
#3899=VECTOR('',#12791,1000.);
#3900=VECTOR('',#12792,1000.);
#3901=VECTOR('',#12793,1000.);
#3902=VECTOR('',#12796,1000.);
#3903=VECTOR('',#12799,1000.);
#3904=VECTOR('',#12804,1000.);
#3905=VECTOR('',#12805,1000.);
#3906=VECTOR('',#12806,1000.);
#3907=VECTOR('',#12809,1000.);
#3908=VECTOR('',#12810,1000.);
#3909=VECTOR('',#12811,1000.);
#3910=VECTOR('',#12814,1000.);
#3911=VECTOR('',#12817,1000.);
#3912=VECTOR('',#12822,1000.);
#3913=VECTOR('',#12823,1000.);
#3914=VECTOR('',#12824,1000.);
#3915=VECTOR('',#12827,1000.);
#3916=VECTOR('',#12828,1000.);
#3917=VECTOR('',#12829,1000.);
#3918=VECTOR('',#12832,1000.);
#3919=VECTOR('',#12835,1000.);
#3920=VECTOR('',#12840,1000.);
#3921=VECTOR('',#12841,1000.);
#3922=VECTOR('',#12842,1000.);
#3923=VECTOR('',#12845,1000.);
#3924=VECTOR('',#12846,1000.);
#3925=VECTOR('',#12847,1000.);
#3926=VECTOR('',#12850,1000.);
#3927=VECTOR('',#12853,1000.);
#3928=VECTOR('',#12858,1000.);
#3929=VECTOR('',#12859,1000.);
#3930=VECTOR('',#12860,1000.);
#3931=VECTOR('',#12863,1000.);
#3932=VECTOR('',#12864,1000.);
#3933=VECTOR('',#12865,1000.);
#3934=VECTOR('',#12868,1000.);
#3935=VECTOR('',#12871,1000.);
#3936=VECTOR('',#12876,1000.);
#3937=VECTOR('',#12877,1000.);
#3938=VECTOR('',#12878,1000.);
#3939=VECTOR('',#12881,1000.);
#3940=VECTOR('',#12882,1000.);
#3941=VECTOR('',#12883,1000.);
#3942=VECTOR('',#12886,1000.);
#3943=VECTOR('',#12889,1000.);
#3944=VECTOR('',#12894,1000.);
#3945=VECTOR('',#12895,1000.);
#3946=VECTOR('',#12896,1000.);
#3947=VECTOR('',#12899,1000.);
#3948=VECTOR('',#12900,1000.);
#3949=VECTOR('',#12901,1000.);
#3950=VECTOR('',#12904,1000.);
#3951=VECTOR('',#12907,1000.);
#3952=VECTOR('',#12912,1000.);
#3953=VECTOR('',#12913,1000.);
#3954=VECTOR('',#12914,1000.);
#3955=VECTOR('',#12917,1000.);
#3956=VECTOR('',#12918,1000.);
#3957=VECTOR('',#12919,1000.);
#3958=VECTOR('',#12922,1000.);
#3959=VECTOR('',#12925,1000.);
#3960=VECTOR('',#12930,1000.);
#3961=VECTOR('',#12931,1000.);
#3962=VECTOR('',#12932,1000.);
#3963=VECTOR('',#12935,1000.);
#3964=VECTOR('',#12936,1000.);
#3965=VECTOR('',#12937,1000.);
#3966=VECTOR('',#12940,1000.);
#3967=VECTOR('',#12943,1000.);
#3968=VECTOR('',#12948,1000.);
#3969=VECTOR('',#12949,1000.);
#3970=VECTOR('',#12950,1000.);
#3971=VECTOR('',#12953,1000.);
#3972=VECTOR('',#12954,1000.);
#3973=VECTOR('',#12955,1000.);
#3974=VECTOR('',#12958,1000.);
#3975=VECTOR('',#12961,1000.);
#3976=VECTOR('',#12966,1000.);
#3977=VECTOR('',#12967,1000.);
#3978=VECTOR('',#12968,1000.);
#3979=VECTOR('',#12971,1000.);
#3980=VECTOR('',#12972,1000.);
#3981=VECTOR('',#12973,1000.);
#3982=VECTOR('',#12976,1000.);
#3983=VECTOR('',#12979,1000.);
#3984=VECTOR('',#12984,1000.);
#3985=VECTOR('',#12985,1000.);
#3986=VECTOR('',#12986,1000.);
#3987=VECTOR('',#12989,1000.);
#3988=VECTOR('',#12990,1000.);
#3989=VECTOR('',#12991,1000.);
#3990=VECTOR('',#12994,1000.);
#3991=VECTOR('',#12997,1000.);
#3992=VECTOR('',#13002,1000.);
#3993=VECTOR('',#13003,1000.);
#3994=VECTOR('',#13004,1000.);
#3995=VECTOR('',#13007,1000.);
#3996=VECTOR('',#13008,1000.);
#3997=VECTOR('',#13009,1000.);
#3998=VECTOR('',#13012,1000.);
#3999=VECTOR('',#13015,1000.);
#4000=VECTOR('',#13020,1000.);
#4001=VECTOR('',#13021,1000.);
#4002=VECTOR('',#13022,1000.);
#4003=VECTOR('',#13025,1000.);
#4004=VECTOR('',#13026,1000.);
#4005=VECTOR('',#13027,1000.);
#4006=VECTOR('',#13030,1000.);
#4007=VECTOR('',#13033,1000.);
#4008=VECTOR('',#13038,1000.);
#4009=VECTOR('',#13039,1000.);
#4010=VECTOR('',#13040,1000.);
#4011=VECTOR('',#13043,1000.);
#4012=VECTOR('',#13044,1000.);
#4013=VECTOR('',#13045,1000.);
#4014=VECTOR('',#13048,1000.);
#4015=VECTOR('',#13051,1000.);
#4016=VECTOR('',#13056,1000.);
#4017=VECTOR('',#13057,1000.);
#4018=VECTOR('',#13058,1000.);
#4019=VECTOR('',#13061,1000.);
#4020=VECTOR('',#13062,1000.);
#4021=VECTOR('',#13063,1000.);
#4022=VECTOR('',#13066,1000.);
#4023=VECTOR('',#13069,1000.);
#4024=VECTOR('',#13074,1000.);
#4025=VECTOR('',#13075,1000.);
#4026=VECTOR('',#13076,1000.);
#4027=VECTOR('',#13079,1000.);
#4028=VECTOR('',#13080,1000.);
#4029=VECTOR('',#13081,1000.);
#4030=VECTOR('',#13084,1000.);
#4031=VECTOR('',#13087,1000.);
#4032=VECTOR('',#13092,1000.);
#4033=VECTOR('',#13093,1000.);
#4034=VECTOR('',#13094,1000.);
#4035=VECTOR('',#13097,1000.);
#4036=VECTOR('',#13098,1000.);
#4037=VECTOR('',#13099,1000.);
#4038=VECTOR('',#13102,1000.);
#4039=VECTOR('',#13105,1000.);
#4040=VECTOR('',#13110,1000.);
#4041=VECTOR('',#13111,1000.);
#4042=VECTOR('',#13112,1000.);
#4043=VECTOR('',#13115,1000.);
#4044=VECTOR('',#13116,1000.);
#4045=VECTOR('',#13117,1000.);
#4046=VECTOR('',#13120,1000.);
#4047=VECTOR('',#13123,1000.);
#4048=VECTOR('',#13128,1000.);
#4049=VECTOR('',#13129,1000.);
#4050=VECTOR('',#13130,1000.);
#4051=VECTOR('',#13133,1000.);
#4052=VECTOR('',#13134,1000.);
#4053=VECTOR('',#13135,1000.);
#4054=VECTOR('',#13138,1000.);
#4055=VECTOR('',#13141,1000.);
#4056=VECTOR('',#13146,1000.);
#4057=VECTOR('',#13147,1000.);
#4058=VECTOR('',#13148,1000.);
#4059=VECTOR('',#13151,1000.);
#4060=VECTOR('',#13152,1000.);
#4061=VECTOR('',#13153,1000.);
#4062=VECTOR('',#13156,1000.);
#4063=VECTOR('',#13159,1000.);
#4064=VECTOR('',#13164,1000.);
#4065=VECTOR('',#13165,1000.);
#4066=VECTOR('',#13166,1000.);
#4067=VECTOR('',#13169,1000.);
#4068=VECTOR('',#13170,1000.);
#4069=VECTOR('',#13171,1000.);
#4070=VECTOR('',#13174,1000.);
#4071=VECTOR('',#13177,1000.);
#4072=VECTOR('',#13182,1000.);
#4073=VECTOR('',#13183,1000.);
#4074=VECTOR('',#13184,1000.);
#4075=VECTOR('',#13187,1000.);
#4076=VECTOR('',#13188,1000.);
#4077=VECTOR('',#13189,1000.);
#4078=VECTOR('',#13192,1000.);
#4079=VECTOR('',#13195,1000.);
#4080=VECTOR('',#13200,1000.);
#4081=VECTOR('',#13201,1000.);
#4082=VECTOR('',#13202,1000.);
#4083=VECTOR('',#13205,1000.);
#4084=VECTOR('',#13206,1000.);
#4085=VECTOR('',#13207,1000.);
#4086=VECTOR('',#13210,1000.);
#4087=VECTOR('',#13213,1000.);
#4088=VECTOR('',#13218,1000.);
#4089=VECTOR('',#13219,1000.);
#4090=VECTOR('',#13220,1000.);
#4091=VECTOR('',#13223,1000.);
#4092=VECTOR('',#13224,1000.);
#4093=VECTOR('',#13225,1000.);
#4094=VECTOR('',#13228,1000.);
#4095=VECTOR('',#13231,1000.);
#4096=VECTOR('',#13236,1000.);
#4097=VECTOR('',#13237,1000.);
#4098=VECTOR('',#13238,1000.);
#4099=VECTOR('',#13241,1000.);
#4100=VECTOR('',#13242,1000.);
#4101=VECTOR('',#13243,1000.);
#4102=VECTOR('',#13246,1000.);
#4103=VECTOR('',#13249,1000.);
#4342=CIRCLE('',#10489,6.2);
#4343=CIRCLE('',#10490,6.2);
#4344=CIRCLE('',#10492,14.);
#4345=CIRCLE('',#10493,14.);
#4346=CIRCLE('',#10494,14.);
#4347=CIRCLE('',#10495,14.);
#4348=CIRCLE('',#10496,14.);
#4349=CIRCLE('',#10497,14.);
#4350=CIRCLE('',#10498,14.);
#4351=CIRCLE('',#10499,14.);
#4352=CIRCLE('',#10500,14.);
#4353=CIRCLE('',#10501,14.);
#4354=CIRCLE('',#10502,14.);
#4355=CIRCLE('',#10503,14.);
#4356=CIRCLE('',#10504,14.);
#4357=CIRCLE('',#10505,14.);
#4358=CIRCLE('',#10506,14.);
#4359=CIRCLE('',#10507,14.);
#4360=CIRCLE('',#10508,14.);
#4361=CIRCLE('',#10509,14.);
#4362=CIRCLE('',#10510,14.);
#4363=CIRCLE('',#10511,14.);
#4364=CIRCLE('',#10512,14.);
#4365=CIRCLE('',#10513,14.);
#4366=CIRCLE('',#10514,14.);
#4367=CIRCLE('',#10515,14.);
#4368=CIRCLE('',#10516,14.);
#4369=CIRCLE('',#10517,14.);
#4370=CIRCLE('',#10518,14.);
#4371=CIRCLE('',#10519,14.);
#4372=CIRCLE('',#10520,14.);
#4373=CIRCLE('',#10521,14.);
#4374=CIRCLE('',#10522,14.);
#4375=CIRCLE('',#10523,14.);
#4376=CIRCLE('',#10524,14.);
#4377=CIRCLE('',#10525,14.);
#4378=CIRCLE('',#10526,14.);
#4379=CIRCLE('',#10527,14.);
#4380=CIRCLE('',#10528,14.);
#4381=CIRCLE('',#10529,14.);
#4382=CIRCLE('',#10530,14.);
#4383=CIRCLE('',#10531,14.);
#4384=CIRCLE('',#10532,14.);
#4385=CIRCLE('',#10533,14.);
#4386=CIRCLE('',#10534,14.);
#4387=CIRCLE('',#10535,14.);
#4388=CIRCLE('',#10536,14.);
#4389=CIRCLE('',#10537,14.);
#4390=CIRCLE('',#10538,14.);
#4391=CIRCLE('',#10539,14.);
#4392=CIRCLE('',#10540,14.);
#4393=CIRCLE('',#10541,14.);
#4394=CIRCLE('',#10542,14.);
#4395=CIRCLE('',#10543,14.);
#4396=CIRCLE('',#10544,14.);
#4397=CIRCLE('',#10545,14.);
#4398=CIRCLE('',#10546,14.);
#4399=CIRCLE('',#10547,14.);
#4400=CIRCLE('',#10548,14.);
#4401=CIRCLE('',#10549,14.);
#4402=CIRCLE('',#10550,14.);
#4403=CIRCLE('',#10551,14.);
#4404=CIRCLE('',#10552,14.);
#4405=CIRCLE('',#10553,14.);
#4406=CIRCLE('',#10554,14.);
#4407=CIRCLE('',#10555,14.);
#4408=CIRCLE('',#10556,14.);
#4409=CIRCLE('',#10557,14.);
#4410=CIRCLE('',#10558,14.);
#4411=CIRCLE('',#10559,14.);
#4412=CIRCLE('',#10560,14.);
#4413=CIRCLE('',#10561,14.);
#4414=CIRCLE('',#10562,14.);
#4415=CIRCLE('',#10563,14.);
#4416=CIRCLE('',#10564,14.);
#4417=CIRCLE('',#10565,14.);
#4418=CIRCLE('',#10566,14.);
#4419=CIRCLE('',#10567,14.);
#4420=CIRCLE('',#10568,14.);
#4421=CIRCLE('',#10569,14.);
#4422=CIRCLE('',#10570,14.);
#4423=CIRCLE('',#10571,14.);
#4424=CIRCLE('',#10572,14.);
#4425=CIRCLE('',#10573,14.);
#4426=CIRCLE('',#10574,14.);
#4427=CIRCLE('',#10575,14.);
#4882=VERTEX_POINT('',#15148);
#4883=VERTEX_POINT('',#15150);
#4884=VERTEX_POINT('',#15154);
#4885=VERTEX_POINT('',#15156);
#4886=VERTEX_POINT('',#15158);
#4887=VERTEX_POINT('',#15160);
#4888=VERTEX_POINT('',#15162);
#4889=VERTEX_POINT('',#15164);
#4890=VERTEX_POINT('',#15167);
#4891=VERTEX_POINT('',#15169);
#4892=VERTEX_POINT('',#15172);
#4893=VERTEX_POINT('',#15173);
#4894=VERTEX_POINT('',#15175);
#4895=VERTEX_POINT('',#15177);
#4896=VERTEX_POINT('',#15180);
#4897=VERTEX_POINT('',#15181);
#4898=VERTEX_POINT('',#15183);
#4899=VERTEX_POINT('',#15185);
#4900=VERTEX_POINT('',#15188);
#4901=VERTEX_POINT('',#15189);
#4902=VERTEX_POINT('',#15191);
#4903=VERTEX_POINT('',#15193);
#4904=VERTEX_POINT('',#15196);
#4905=VERTEX_POINT('',#15197);
#4906=VERTEX_POINT('',#15199);
#4907=VERTEX_POINT('',#15201);
#4908=VERTEX_POINT('',#15204);
#4909=VERTEX_POINT('',#15205);
#4910=VERTEX_POINT('',#15207);
#4911=VERTEX_POINT('',#15209);
#4912=VERTEX_POINT('',#15212);
#4913=VERTEX_POINT('',#15213);
#4914=VERTEX_POINT('',#15215);
#4915=VERTEX_POINT('',#15217);
#4916=VERTEX_POINT('',#15220);
#4917=VERTEX_POINT('',#15221);
#4918=VERTEX_POINT('',#15223);
#4919=VERTEX_POINT('',#15225);
#4920=VERTEX_POINT('',#15228);
#4921=VERTEX_POINT('',#15229);
#4922=VERTEX_POINT('',#15231);
#4923=VERTEX_POINT('',#15233);
#4924=VERTEX_POINT('',#15236);
#4925=VERTEX_POINT('',#15237);
#4926=VERTEX_POINT('',#15239);
#4927=VERTEX_POINT('',#15241);
#4928=VERTEX_POINT('',#15244);
#4929=VERTEX_POINT('',#15245);
#4930=VERTEX_POINT('',#15247);
#4931=VERTEX_POINT('',#15249);
#4932=VERTEX_POINT('',#15252);
#4933=VERTEX_POINT('',#15253);
#4934=VERTEX_POINT('',#15255);
#4935=VERTEX_POINT('',#15257);
#4936=VERTEX_POINT('',#15260);
#4937=VERTEX_POINT('',#15261);
#4938=VERTEX_POINT('',#15263);
#4939=VERTEX_POINT('',#15265);
#4940=VERTEX_POINT('',#15268);
#4941=VERTEX_POINT('',#15269);
#4942=VERTEX_POINT('',#15271);
#4943=VERTEX_POINT('',#15273);
#4944=VERTEX_POINT('',#15276);
#4945=VERTEX_POINT('',#15277);
#4946=VERTEX_POINT('',#15279);
#4947=VERTEX_POINT('',#15281);
#4948=VERTEX_POINT('',#15284);
#4949=VERTEX_POINT('',#15285);
#4950=VERTEX_POINT('',#15287);
#4951=VERTEX_POINT('',#15289);
#4952=VERTEX_POINT('',#15292);
#4953=VERTEX_POINT('',#15293);
#4954=VERTEX_POINT('',#15295);
#4955=VERTEX_POINT('',#15297);
#4956=VERTEX_POINT('',#15300);
#4957=VERTEX_POINT('',#15301);
#4958=VERTEX_POINT('',#15303);
#4959=VERTEX_POINT('',#15305);
#4960=VERTEX_POINT('',#15308);
#4961=VERTEX_POINT('',#15309);
#4962=VERTEX_POINT('',#15311);
#4963=VERTEX_POINT('',#15313);
#4964=VERTEX_POINT('',#15316);
#4965=VERTEX_POINT('',#15317);
#4966=VERTEX_POINT('',#15319);
#4967=VERTEX_POINT('',#15321);
#4968=VERTEX_POINT('',#15324);
#4969=VERTEX_POINT('',#15325);
#4970=VERTEX_POINT('',#15327);
#4971=VERTEX_POINT('',#15329);
#4972=VERTEX_POINT('',#15332);
#4973=VERTEX_POINT('',#15333);
#4974=VERTEX_POINT('',#15335);
#4975=VERTEX_POINT('',#15337);
#4976=VERTEX_POINT('',#15340);
#4977=VERTEX_POINT('',#15341);
#4978=VERTEX_POINT('',#15343);
#4979=VERTEX_POINT('',#15345);
#4980=VERTEX_POINT('',#15348);
#4981=VERTEX_POINT('',#15349);
#4982=VERTEX_POINT('',#15351);
#4983=VERTEX_POINT('',#15353);
#4984=VERTEX_POINT('',#15356);
#4985=VERTEX_POINT('',#15357);
#4986=VERTEX_POINT('',#15359);
#4987=VERTEX_POINT('',#15361);
#4988=VERTEX_POINT('',#15364);
#4989=VERTEX_POINT('',#15365);
#4990=VERTEX_POINT('',#15367);
#4991=VERTEX_POINT('',#15369);
#4992=VERTEX_POINT('',#15372);
#4993=VERTEX_POINT('',#15373);
#4994=VERTEX_POINT('',#15375);
#4995=VERTEX_POINT('',#15377);
#4996=VERTEX_POINT('',#15380);
#4997=VERTEX_POINT('',#15381);
#4998=VERTEX_POINT('',#15383);
#4999=VERTEX_POINT('',#15385);
#5000=VERTEX_POINT('',#15388);
#5001=VERTEX_POINT('',#15389);
#5002=VERTEX_POINT('',#15391);
#5003=VERTEX_POINT('',#15393);
#5004=VERTEX_POINT('',#15396);
#5005=VERTEX_POINT('',#15397);
#5006=VERTEX_POINT('',#15399);
#5007=VERTEX_POINT('',#15401);
#5008=VERTEX_POINT('',#15404);
#5009=VERTEX_POINT('',#15405);
#5010=VERTEX_POINT('',#15407);
#5011=VERTEX_POINT('',#15409);
#5012=VERTEX_POINT('',#15412);
#5013=VERTEX_POINT('',#15413);
#5014=VERTEX_POINT('',#15415);
#5015=VERTEX_POINT('',#15417);
#5016=VERTEX_POINT('',#15420);
#5017=VERTEX_POINT('',#15421);
#5018=VERTEX_POINT('',#15423);
#5019=VERTEX_POINT('',#15425);
#5020=VERTEX_POINT('',#15428);
#5021=VERTEX_POINT('',#15429);
#5022=VERTEX_POINT('',#15431);
#5023=VERTEX_POINT('',#15433);
#5024=VERTEX_POINT('',#15436);
#5025=VERTEX_POINT('',#15437);
#5026=VERTEX_POINT('',#15439);
#5027=VERTEX_POINT('',#15441);
#5028=VERTEX_POINT('',#15444);
#5029=VERTEX_POINT('',#15445);
#5030=VERTEX_POINT('',#15447);
#5031=VERTEX_POINT('',#15449);
#5032=VERTEX_POINT('',#15452);
#5033=VERTEX_POINT('',#15453);
#5034=VERTEX_POINT('',#15455);
#5035=VERTEX_POINT('',#15457);
#5036=VERTEX_POINT('',#15460);
#5037=VERTEX_POINT('',#15461);
#5038=VERTEX_POINT('',#15463);
#5039=VERTEX_POINT('',#15465);
#5040=VERTEX_POINT('',#15468);
#5041=VERTEX_POINT('',#15469);
#5042=VERTEX_POINT('',#15471);
#5043=VERTEX_POINT('',#15473);
#5044=VERTEX_POINT('',#15476);
#5045=VERTEX_POINT('',#15477);
#5046=VERTEX_POINT('',#15479);
#5047=VERTEX_POINT('',#15481);
#5048=VERTEX_POINT('',#15487);
#5049=VERTEX_POINT('',#15489);
#5050=VERTEX_POINT('',#15493);
#5051=VERTEX_POINT('',#15495);
#5052=VERTEX_POINT('',#15504);
#5053=VERTEX_POINT('',#15506);
#5054=VERTEX_POINT('',#15510);
#5055=VERTEX_POINT('',#15512);
#5056=VERTEX_POINT('',#15521);
#5057=VERTEX_POINT('',#15523);
#5058=VERTEX_POINT('',#15527);
#5059=VERTEX_POINT('',#15529);
#5060=VERTEX_POINT('',#15538);
#5061=VERTEX_POINT('',#15540);
#5062=VERTEX_POINT('',#15544);
#5063=VERTEX_POINT('',#15546);
#5064=VERTEX_POINT('',#15555);
#5065=VERTEX_POINT('',#15557);
#5066=VERTEX_POINT('',#15561);
#5067=VERTEX_POINT('',#15563);
#5068=VERTEX_POINT('',#15572);
#5069=VERTEX_POINT('',#15574);
#5070=VERTEX_POINT('',#15578);
#5071=VERTEX_POINT('',#15580);
#5072=VERTEX_POINT('',#15589);
#5073=VERTEX_POINT('',#15591);
#5074=VERTEX_POINT('',#15595);
#5075=VERTEX_POINT('',#15597);
#5076=VERTEX_POINT('',#15606);
#5077=VERTEX_POINT('',#15608);
#5078=VERTEX_POINT('',#15612);
#5079=VERTEX_POINT('',#15614);
#5080=VERTEX_POINT('',#15623);
#5081=VERTEX_POINT('',#15625);
#5082=VERTEX_POINT('',#15629);
#5083=VERTEX_POINT('',#15631);
#5084=VERTEX_POINT('',#15640);
#5085=VERTEX_POINT('',#15642);
#5086=VERTEX_POINT('',#15646);
#5087=VERTEX_POINT('',#15648);
#5088=VERTEX_POINT('',#15657);
#5089=VERTEX_POINT('',#15659);
#5090=VERTEX_POINT('',#15663);
#5091=VERTEX_POINT('',#15665);
#5092=VERTEX_POINT('',#15674);
#5093=VERTEX_POINT('',#15676);
#5094=VERTEX_POINT('',#15680);
#5095=VERTEX_POINT('',#15682);
#5096=VERTEX_POINT('',#15691);
#5097=VERTEX_POINT('',#15693);
#5098=VERTEX_POINT('',#15697);
#5099=VERTEX_POINT('',#15699);
#5100=VERTEX_POINT('',#15708);
#5101=VERTEX_POINT('',#15710);
#5102=VERTEX_POINT('',#15714);
#5103=VERTEX_POINT('',#15716);
#5104=VERTEX_POINT('',#15725);
#5105=VERTEX_POINT('',#15727);
#5106=VERTEX_POINT('',#15731);
#5107=VERTEX_POINT('',#15733);
#5108=VERTEX_POINT('',#15742);
#5109=VERTEX_POINT('',#15744);
#5110=VERTEX_POINT('',#15748);
#5111=VERTEX_POINT('',#15750);
#5112=VERTEX_POINT('',#15759);
#5113=VERTEX_POINT('',#15761);
#5114=VERTEX_POINT('',#15765);
#5115=VERTEX_POINT('',#15767);
#5116=VERTEX_POINT('',#15776);
#5117=VERTEX_POINT('',#15778);
#5118=VERTEX_POINT('',#15782);
#5119=VERTEX_POINT('',#15784);
#5120=VERTEX_POINT('',#15793);
#5121=VERTEX_POINT('',#15795);
#5122=VERTEX_POINT('',#15799);
#5123=VERTEX_POINT('',#15801);
#5124=VERTEX_POINT('',#15810);
#5125=VERTEX_POINT('',#15812);
#5126=VERTEX_POINT('',#15816);
#5127=VERTEX_POINT('',#15818);
#5128=VERTEX_POINT('',#15827);
#5129=VERTEX_POINT('',#15829);
#5130=VERTEX_POINT('',#15833);
#5131=VERTEX_POINT('',#15835);
#5132=VERTEX_POINT('',#15844);
#5133=VERTEX_POINT('',#15846);
#5134=VERTEX_POINT('',#15850);
#5135=VERTEX_POINT('',#15852);
#5136=VERTEX_POINT('',#15861);
#5137=VERTEX_POINT('',#15863);
#5138=VERTEX_POINT('',#15867);
#5139=VERTEX_POINT('',#15869);
#5140=VERTEX_POINT('',#15878);
#5141=VERTEX_POINT('',#15880);
#5142=VERTEX_POINT('',#15884);
#5143=VERTEX_POINT('',#15886);
#5144=VERTEX_POINT('',#15895);
#5145=VERTEX_POINT('',#15897);
#5146=VERTEX_POINT('',#15901);
#5147=VERTEX_POINT('',#15903);
#5148=VERTEX_POINT('',#15912);
#5149=VERTEX_POINT('',#15914);
#5150=VERTEX_POINT('',#15918);
#5151=VERTEX_POINT('',#15920);
#5152=VERTEX_POINT('',#15929);
#5153=VERTEX_POINT('',#15931);
#5154=VERTEX_POINT('',#15935);
#5155=VERTEX_POINT('',#15937);
#5156=VERTEX_POINT('',#15946);
#5157=VERTEX_POINT('',#15948);
#5158=VERTEX_POINT('',#15952);
#5159=VERTEX_POINT('',#15954);
#5160=VERTEX_POINT('',#15963);
#5161=VERTEX_POINT('',#15965);
#5162=VERTEX_POINT('',#15969);
#5163=VERTEX_POINT('',#15971);
#5164=VERTEX_POINT('',#15980);
#5165=VERTEX_POINT('',#15982);
#5166=VERTEX_POINT('',#15986);
#5167=VERTEX_POINT('',#15988);
#5168=VERTEX_POINT('',#15997);
#5169=VERTEX_POINT('',#15999);
#5170=VERTEX_POINT('',#16003);
#5171=VERTEX_POINT('',#16005);
#5172=VERTEX_POINT('',#16014);
#5173=VERTEX_POINT('',#16016);
#5174=VERTEX_POINT('',#16020);
#5175=VERTEX_POINT('',#16022);
#5176=VERTEX_POINT('',#16031);
#5177=VERTEX_POINT('',#16033);
#5178=VERTEX_POINT('',#16037);
#5179=VERTEX_POINT('',#16039);
#5180=VERTEX_POINT('',#16048);
#5181=VERTEX_POINT('',#16050);
#5182=VERTEX_POINT('',#16054);
#5183=VERTEX_POINT('',#16056);
#5184=VERTEX_POINT('',#16065);
#5185=VERTEX_POINT('',#16067);
#5186=VERTEX_POINT('',#16071);
#5187=VERTEX_POINT('',#16073);
#5188=VERTEX_POINT('',#16082);
#5189=VERTEX_POINT('',#16084);
#5190=VERTEX_POINT('',#16088);
#5191=VERTEX_POINT('',#16090);
#5192=VERTEX_POINT('',#16099);
#5193=VERTEX_POINT('',#16101);
#5194=VERTEX_POINT('',#16105);
#5195=VERTEX_POINT('',#16107);
#5196=VERTEX_POINT('',#16116);
#5197=VERTEX_POINT('',#16118);
#5198=VERTEX_POINT('',#16122);
#5199=VERTEX_POINT('',#16124);
#5200=VERTEX_POINT('',#16133);
#5201=VERTEX_POINT('',#16135);
#5202=VERTEX_POINT('',#16139);
#5203=VERTEX_POINT('',#16141);
#5204=VERTEX_POINT('',#16150);
#5205=VERTEX_POINT('',#16152);
#5206=VERTEX_POINT('',#16156);
#5207=VERTEX_POINT('',#16158);
#5953=EDGE_CURVE('',#4882,#4882,#4342,.T.);
#5954=EDGE_CURVE('',#4882,#4883,#2653,.T.);
#5955=EDGE_CURVE('',#4883,#4883,#4343,.T.);
#5956=EDGE_CURVE('',#4884,#4884,#4344,.T.);
#5957=EDGE_CURVE('',#4884,#4885,#2654,.T.);
#5958=EDGE_CURVE('',#4886,#4885,#4345,.T.);
#5959=EDGE_CURVE('',#4887,#4886,#2655,.T.);
#5960=EDGE_CURVE('',#4887,#4888,#4346,.T.);
#5961=EDGE_CURVE('',#4888,#4889,#2656,.T.);
#5962=EDGE_CURVE('',#4889,#4889,#4347,.T.);
#5963=EDGE_CURVE('',#4888,#4890,#4348,.T.);
#5964=EDGE_CURVE('',#4891,#4890,#2657,.T.);
#5965=EDGE_CURVE('',#4885,#4891,#4349,.T.);
#5966=EDGE_CURVE('',#4892,#4893,#4350,.T.);
#5967=EDGE_CURVE('',#4894,#4893,#2658,.T.);
#5968=EDGE_CURVE('',#4895,#4894,#4351,.T.);
#5969=EDGE_CURVE('',#4892,#4895,#2659,.T.);
#5970=EDGE_CURVE('',#4896,#4897,#2660,.T.);
#5971=EDGE_CURVE('',#4896,#4898,#4352,.T.);
#5972=EDGE_CURVE('',#4899,#4898,#2661,.T.);
#5973=EDGE_CURVE('',#4897,#4899,#4353,.T.);
#5974=EDGE_CURVE('',#4900,#4901,#2662,.T.);
#5975=EDGE_CURVE('',#4900,#4902,#4354,.T.);
#5976=EDGE_CURVE('',#4903,#4902,#2663,.T.);
#5977=EDGE_CURVE('',#4901,#4903,#4355,.T.);
#5978=EDGE_CURVE('',#4904,#4905,#2664,.T.);
#5979=EDGE_CURVE('',#4904,#4906,#4356,.T.);
#5980=EDGE_CURVE('',#4907,#4906,#2665,.T.);
#5981=EDGE_CURVE('',#4905,#4907,#4357,.T.);
#5982=EDGE_CURVE('',#4908,#4909,#2666,.T.);
#5983=EDGE_CURVE('',#4908,#4910,#4358,.T.);
#5984=EDGE_CURVE('',#4911,#4910,#2667,.T.);
#5985=EDGE_CURVE('',#4909,#4911,#4359,.T.);
#5986=EDGE_CURVE('',#4912,#4913,#2668,.T.);
#5987=EDGE_CURVE('',#4912,#4914,#4360,.T.);
#5988=EDGE_CURVE('',#4915,#4914,#2669,.T.);
#5989=EDGE_CURVE('',#4913,#4915,#4361,.T.);
#5990=EDGE_CURVE('',#4916,#4917,#2670,.T.);
#5991=EDGE_CURVE('',#4916,#4918,#4362,.T.);
#5992=EDGE_CURVE('',#4919,#4918,#2671,.T.);
#5993=EDGE_CURVE('',#4917,#4919,#4363,.T.);
#5994=EDGE_CURVE('',#4920,#4921,#2672,.T.);
#5995=EDGE_CURVE('',#4920,#4922,#4364,.T.);
#5996=EDGE_CURVE('',#4923,#4922,#2673,.T.);
#5997=EDGE_CURVE('',#4921,#4923,#4365,.T.);
#5998=EDGE_CURVE('',#4924,#4925,#2674,.T.);
#5999=EDGE_CURVE('',#4924,#4926,#4366,.T.);
#6000=EDGE_CURVE('',#4927,#4926,#2675,.T.);
#6001=EDGE_CURVE('',#4925,#4927,#4367,.T.);
#6002=EDGE_CURVE('',#4928,#4929,#2676,.T.);
#6003=EDGE_CURVE('',#4928,#4930,#4368,.T.);
#6004=EDGE_CURVE('',#4931,#4930,#2677,.T.);
#6005=EDGE_CURVE('',#4929,#4931,#4369,.T.);
#6006=EDGE_CURVE('',#4932,#4933,#2678,.T.);
#6007=EDGE_CURVE('',#4932,#4934,#4370,.T.);
#6008=EDGE_CURVE('',#4935,#4934,#2679,.T.);
#6009=EDGE_CURVE('',#4933,#4935,#4371,.T.);
#6010=EDGE_CURVE('',#4936,#4937,#2680,.T.);
#6011=EDGE_CURVE('',#4936,#4938,#4372,.T.);
#6012=EDGE_CURVE('',#4939,#4938,#2681,.T.);
#6013=EDGE_CURVE('',#4937,#4939,#4373,.T.);
#6014=EDGE_CURVE('',#4940,#4941,#2682,.T.);
#6015=EDGE_CURVE('',#4940,#4942,#4374,.T.);
#6016=EDGE_CURVE('',#4943,#4942,#2683,.T.);
#6017=EDGE_CURVE('',#4941,#4943,#4375,.T.);
#6018=EDGE_CURVE('',#4944,#4945,#2684,.T.);
#6019=EDGE_CURVE('',#4944,#4946,#4376,.T.);
#6020=EDGE_CURVE('',#4947,#4946,#2685,.T.);
#6021=EDGE_CURVE('',#4945,#4947,#4377,.T.);
#6022=EDGE_CURVE('',#4948,#4949,#2686,.T.);
#6023=EDGE_CURVE('',#4948,#4950,#4378,.T.);
#6024=EDGE_CURVE('',#4951,#4950,#2687,.T.);
#6025=EDGE_CURVE('',#4949,#4951,#4379,.T.);
#6026=EDGE_CURVE('',#4952,#4953,#2688,.T.);
#6027=EDGE_CURVE('',#4952,#4954,#4380,.T.);
#6028=EDGE_CURVE('',#4955,#4954,#2689,.T.);
#6029=EDGE_CURVE('',#4953,#4955,#4381,.T.);
#6030=EDGE_CURVE('',#4956,#4957,#2690,.T.);
#6031=EDGE_CURVE('',#4956,#4958,#4382,.T.);
#6032=EDGE_CURVE('',#4959,#4958,#2691,.T.);
#6033=EDGE_CURVE('',#4957,#4959,#4383,.T.);
#6034=EDGE_CURVE('',#4960,#4961,#2692,.T.);
#6035=EDGE_CURVE('',#4960,#4962,#4384,.T.);
#6036=EDGE_CURVE('',#4963,#4962,#2693,.T.);
#6037=EDGE_CURVE('',#4961,#4963,#4385,.T.);
#6038=EDGE_CURVE('',#4964,#4965,#2694,.T.);
#6039=EDGE_CURVE('',#4964,#4966,#4386,.T.);
#6040=EDGE_CURVE('',#4967,#4966,#2695,.T.);
#6041=EDGE_CURVE('',#4965,#4967,#4387,.T.);
#6042=EDGE_CURVE('',#4968,#4969,#2696,.T.);
#6043=EDGE_CURVE('',#4968,#4970,#4388,.T.);
#6044=EDGE_CURVE('',#4971,#4970,#2697,.T.);
#6045=EDGE_CURVE('',#4969,#4971,#4389,.T.);
#6046=EDGE_CURVE('',#4972,#4973,#2698,.T.);
#6047=EDGE_CURVE('',#4972,#4974,#4390,.T.);
#6048=EDGE_CURVE('',#4975,#4974,#2699,.T.);
#6049=EDGE_CURVE('',#4973,#4975,#4391,.T.);
#6050=EDGE_CURVE('',#4976,#4977,#2700,.T.);
#6051=EDGE_CURVE('',#4976,#4978,#4392,.T.);
#6052=EDGE_CURVE('',#4979,#4978,#2701,.T.);
#6053=EDGE_CURVE('',#4977,#4979,#4393,.T.);
#6054=EDGE_CURVE('',#4980,#4981,#2702,.T.);
#6055=EDGE_CURVE('',#4980,#4982,#4394,.T.);
#6056=EDGE_CURVE('',#4983,#4982,#2703,.T.);
#6057=EDGE_CURVE('',#4981,#4983,#4395,.T.);
#6058=EDGE_CURVE('',#4984,#4985,#2704,.T.);
#6059=EDGE_CURVE('',#4984,#4986,#4396,.T.);
#6060=EDGE_CURVE('',#4987,#4986,#2705,.T.);
#6061=EDGE_CURVE('',#4985,#4987,#4397,.T.);
#6062=EDGE_CURVE('',#4988,#4989,#2706,.T.);
#6063=EDGE_CURVE('',#4988,#4990,#4398,.T.);
#6064=EDGE_CURVE('',#4991,#4990,#2707,.T.);
#6065=EDGE_CURVE('',#4989,#4991,#4399,.T.);
#6066=EDGE_CURVE('',#4992,#4993,#2708,.T.);
#6067=EDGE_CURVE('',#4992,#4994,#4400,.T.);
#6068=EDGE_CURVE('',#4995,#4994,#2709,.T.);
#6069=EDGE_CURVE('',#4993,#4995,#4401,.T.);
#6070=EDGE_CURVE('',#4996,#4997,#2710,.T.);
#6071=EDGE_CURVE('',#4996,#4998,#4402,.T.);
#6072=EDGE_CURVE('',#4999,#4998,#2711,.T.);
#6073=EDGE_CURVE('',#4997,#4999,#4403,.T.);
#6074=EDGE_CURVE('',#5000,#5001,#2712,.T.);
#6075=EDGE_CURVE('',#5000,#5002,#4404,.T.);
#6076=EDGE_CURVE('',#5003,#5002,#2713,.T.);
#6077=EDGE_CURVE('',#5001,#5003,#4405,.T.);
#6078=EDGE_CURVE('',#5004,#5005,#2714,.T.);
#6079=EDGE_CURVE('',#5004,#5006,#4406,.T.);
#6080=EDGE_CURVE('',#5007,#5006,#2715,.T.);
#6081=EDGE_CURVE('',#5005,#5007,#4407,.T.);
#6082=EDGE_CURVE('',#5008,#5009,#2716,.T.);
#6083=EDGE_CURVE('',#5008,#5010,#4408,.T.);
#6084=EDGE_CURVE('',#5011,#5010,#2717,.T.);
#6085=EDGE_CURVE('',#5009,#5011,#4409,.T.);
#6086=EDGE_CURVE('',#5012,#5013,#2718,.T.);
#6087=EDGE_CURVE('',#5012,#5014,#4410,.T.);
#6088=EDGE_CURVE('',#5015,#5014,#2719,.T.);
#6089=EDGE_CURVE('',#5013,#5015,#4411,.T.);
#6090=EDGE_CURVE('',#5016,#5017,#2720,.T.);
#6091=EDGE_CURVE('',#5016,#5018,#4412,.T.);
#6092=EDGE_CURVE('',#5019,#5018,#2721,.T.);
#6093=EDGE_CURVE('',#5017,#5019,#4413,.T.);
#6094=EDGE_CURVE('',#5020,#5021,#2722,.T.);
#6095=EDGE_CURVE('',#5020,#5022,#4414,.T.);
#6096=EDGE_CURVE('',#5023,#5022,#2723,.T.);
#6097=EDGE_CURVE('',#5021,#5023,#4415,.T.);
#6098=EDGE_CURVE('',#5024,#5025,#2724,.T.);
#6099=EDGE_CURVE('',#5024,#5026,#4416,.T.);
#6100=EDGE_CURVE('',#5027,#5026,#2725,.T.);
#6101=EDGE_CURVE('',#5025,#5027,#4417,.T.);
#6102=EDGE_CURVE('',#5028,#5029,#2726,.T.);
#6103=EDGE_CURVE('',#5028,#5030,#4418,.T.);
#6104=EDGE_CURVE('',#5031,#5030,#2727,.T.);
#6105=EDGE_CURVE('',#5029,#5031,#4419,.T.);
#6106=EDGE_CURVE('',#5032,#5033,#2728,.T.);
#6107=EDGE_CURVE('',#5032,#5034,#4420,.T.);
#6108=EDGE_CURVE('',#5035,#5034,#2729,.T.);
#6109=EDGE_CURVE('',#5033,#5035,#4421,.T.);
#6110=EDGE_CURVE('',#5036,#5037,#2730,.T.);
#6111=EDGE_CURVE('',#5036,#5038,#4422,.T.);
#6112=EDGE_CURVE('',#5039,#5038,#2731,.T.);
#6113=EDGE_CURVE('',#5037,#5039,#4423,.T.);
#6114=EDGE_CURVE('',#5040,#5041,#2732,.T.);
#6115=EDGE_CURVE('',#5040,#5042,#4424,.T.);
#6116=EDGE_CURVE('',#5043,#5042,#2733,.T.);
#6117=EDGE_CURVE('',#5041,#5043,#4425,.T.);
#6118=EDGE_CURVE('',#5044,#5045,#2734,.T.);
#6119=EDGE_CURVE('',#5044,#5046,#4426,.T.);
#6120=EDGE_CURVE('',#5047,#5046,#2735,.T.);
#6121=EDGE_CURVE('',#5045,#5047,#4427,.T.);
#6122=EDGE_CURVE('',#5048,#4897,#2736,.T.);
#6123=EDGE_CURVE('',#5049,#5048,#2737,.T.);
#6124=EDGE_CURVE('',#5049,#4896,#2738,.T.);
#6125=EDGE_CURVE('',#4898,#5050,#2739,.T.);
#6126=EDGE_CURVE('',#5050,#5051,#2740,.T.);
#6127=EDGE_CURVE('',#4899,#5051,#2741,.T.);
#6128=EDGE_CURVE('',#5050,#5049,#2742,.T.);
#6129=EDGE_CURVE('',#5051,#5048,#2743,.T.);
#6130=EDGE_CURVE('',#5052,#4901,#2744,.T.);
#6131=EDGE_CURVE('',#5053,#5052,#2745,.T.);
#6132=EDGE_CURVE('',#5053,#4900,#2746,.T.);
#6133=EDGE_CURVE('',#4902,#5054,#2747,.T.);
#6134=EDGE_CURVE('',#5054,#5055,#2748,.T.);
#6135=EDGE_CURVE('',#4903,#5055,#2749,.T.);
#6136=EDGE_CURVE('',#5054,#5053,#2750,.T.);
#6137=EDGE_CURVE('',#5055,#5052,#2751,.T.);
#6138=EDGE_CURVE('',#5056,#4905,#2752,.T.);
#6139=EDGE_CURVE('',#5057,#5056,#2753,.T.);
#6140=EDGE_CURVE('',#5057,#4904,#2754,.T.);
#6141=EDGE_CURVE('',#4906,#5058,#2755,.T.);
#6142=EDGE_CURVE('',#5058,#5059,#2756,.T.);
#6143=EDGE_CURVE('',#4907,#5059,#2757,.T.);
#6144=EDGE_CURVE('',#5058,#5057,#2758,.T.);
#6145=EDGE_CURVE('',#5059,#5056,#2759,.T.);
#6146=EDGE_CURVE('',#5060,#4895,#2760,.T.);
#6147=EDGE_CURVE('',#5061,#5060,#2761,.T.);
#6148=EDGE_CURVE('',#5061,#4892,#2762,.T.);
#6149=EDGE_CURVE('',#4893,#5062,#2763,.T.);
#6150=EDGE_CURVE('',#5062,#5063,#2764,.T.);
#6151=EDGE_CURVE('',#4894,#5063,#2765,.T.);
#6152=EDGE_CURVE('',#5062,#5061,#2766,.T.);
#6153=EDGE_CURVE('',#5063,#5060,#2767,.T.);
#6154=EDGE_CURVE('',#5064,#4973,#2768,.T.);
#6155=EDGE_CURVE('',#5065,#5064,#2769,.T.);
#6156=EDGE_CURVE('',#5065,#4972,#2770,.T.);
#6157=EDGE_CURVE('',#4974,#5066,#2771,.T.);
#6158=EDGE_CURVE('',#5066,#5067,#2772,.T.);
#6159=EDGE_CURVE('',#4975,#5067,#2773,.T.);
#6160=EDGE_CURVE('',#5066,#5065,#2774,.T.);
#6161=EDGE_CURVE('',#5067,#5064,#2775,.T.);
#6162=EDGE_CURVE('',#5068,#4977,#2776,.T.);
#6163=EDGE_CURVE('',#5069,#5068,#2777,.T.);
#6164=EDGE_CURVE('',#5069,#4976,#2778,.T.);
#6165=EDGE_CURVE('',#4978,#5070,#2779,.T.);
#6166=EDGE_CURVE('',#5070,#5071,#2780,.T.);
#6167=EDGE_CURVE('',#4979,#5071,#2781,.T.);
#6168=EDGE_CURVE('',#5070,#5069,#2782,.T.);
#6169=EDGE_CURVE('',#5071,#5068,#2783,.T.);
#6170=EDGE_CURVE('',#5072,#4981,#2784,.T.);
#6171=EDGE_CURVE('',#5073,#5072,#2785,.T.);
#6172=EDGE_CURVE('',#5073,#4980,#2786,.T.);
#6173=EDGE_CURVE('',#4982,#5074,#2787,.T.);
#6174=EDGE_CURVE('',#5074,#5075,#2788,.T.);
#6175=EDGE_CURVE('',#4983,#5075,#2789,.T.);
#6176=EDGE_CURVE('',#5074,#5073,#2790,.T.);
#6177=EDGE_CURVE('',#5075,#5072,#2791,.T.);
#6178=EDGE_CURVE('',#5076,#4886,#2792,.T.);
#6179=EDGE_CURVE('',#5077,#5076,#2793,.T.);
#6180=EDGE_CURVE('',#5077,#4887,#2794,.T.);
#6181=EDGE_CURVE('',#4890,#5078,#2795,.T.);
#6182=EDGE_CURVE('',#5078,#5079,#2796,.T.);
#6183=EDGE_CURVE('',#4891,#5079,#2797,.T.);
#6184=EDGE_CURVE('',#5078,#5077,#2798,.T.);
#6185=EDGE_CURVE('',#5079,#5076,#2799,.T.);
#6186=EDGE_CURVE('',#5080,#4985,#2800,.T.);
#6187=EDGE_CURVE('',#5081,#5080,#2801,.T.);
#6188=EDGE_CURVE('',#5081,#4984,#2802,.T.);
#6189=EDGE_CURVE('',#4986,#5082,#2803,.T.);
#6190=EDGE_CURVE('',#5082,#5083,#2804,.T.);
#6191=EDGE_CURVE('',#4987,#5083,#2805,.T.);
#6192=EDGE_CURVE('',#5082,#5081,#2806,.T.);
#6193=EDGE_CURVE('',#5083,#5080,#2807,.T.);
#6194=EDGE_CURVE('',#5084,#4909,#2808,.T.);
#6195=EDGE_CURVE('',#5085,#5084,#2809,.T.);
#6196=EDGE_CURVE('',#5085,#4908,#2810,.T.);
#6197=EDGE_CURVE('',#4910,#5086,#2811,.T.);
#6198=EDGE_CURVE('',#5086,#5087,#2812,.T.);
#6199=EDGE_CURVE('',#4911,#5087,#2813,.T.);
#6200=EDGE_CURVE('',#5086,#5085,#2814,.T.);
#6201=EDGE_CURVE('',#5087,#5084,#2815,.T.);
#6202=EDGE_CURVE('',#5088,#4913,#2816,.T.);
#6203=EDGE_CURVE('',#5089,#5088,#2817,.T.);
#6204=EDGE_CURVE('',#5089,#4912,#2818,.T.);
#6205=EDGE_CURVE('',#4914,#5090,#2819,.T.);
#6206=EDGE_CURVE('',#5090,#5091,#2820,.T.);
#6207=EDGE_CURVE('',#4915,#5091,#2821,.T.);
#6208=EDGE_CURVE('',#5090,#5089,#2822,.T.);
#6209=EDGE_CURVE('',#5091,#5088,#2823,.T.);
#6210=EDGE_CURVE('',#5092,#4917,#2824,.T.);
#6211=EDGE_CURVE('',#5093,#5092,#2825,.T.);
#6212=EDGE_CURVE('',#5093,#4916,#2826,.T.);
#6213=EDGE_CURVE('',#4918,#5094,#2827,.T.);
#6214=EDGE_CURVE('',#5094,#5095,#2828,.T.);
#6215=EDGE_CURVE('',#4919,#5095,#2829,.T.);
#6216=EDGE_CURVE('',#5094,#5093,#2830,.T.);
#6217=EDGE_CURVE('',#5095,#5092,#2831,.T.);
#6218=EDGE_CURVE('',#5096,#4921,#2832,.T.);
#6219=EDGE_CURVE('',#5097,#5096,#2833,.T.);
#6220=EDGE_CURVE('',#5097,#4920,#2834,.T.);
#6221=EDGE_CURVE('',#4922,#5098,#2835,.T.);
#6222=EDGE_CURVE('',#5098,#5099,#2836,.T.);
#6223=EDGE_CURVE('',#4923,#5099,#2837,.T.);
#6224=EDGE_CURVE('',#5098,#5097,#2838,.T.);
#6225=EDGE_CURVE('',#5099,#5096,#2839,.T.);
#6226=EDGE_CURVE('',#5100,#4925,#2840,.T.);
#6227=EDGE_CURVE('',#5101,#5100,#2841,.T.);
#6228=EDGE_CURVE('',#5101,#4924,#2842,.T.);
#6229=EDGE_CURVE('',#4926,#5102,#2843,.T.);
#6230=EDGE_CURVE('',#5102,#5103,#2844,.T.);
#6231=EDGE_CURVE('',#4927,#5103,#2845,.T.);
#6232=EDGE_CURVE('',#5102,#5101,#2846,.T.);
#6233=EDGE_CURVE('',#5103,#5100,#2847,.T.);
#6234=EDGE_CURVE('',#5104,#4929,#2848,.T.);
#6235=EDGE_CURVE('',#5105,#5104,#2849,.T.);
#6236=EDGE_CURVE('',#5105,#4928,#2850,.T.);
#6237=EDGE_CURVE('',#4930,#5106,#2851,.T.);
#6238=EDGE_CURVE('',#5106,#5107,#2852,.T.);
#6239=EDGE_CURVE('',#4931,#5107,#2853,.T.);
#6240=EDGE_CURVE('',#5106,#5105,#2854,.T.);
#6241=EDGE_CURVE('',#5107,#5104,#2855,.T.);
#6242=EDGE_CURVE('',#5108,#4933,#2856,.T.);
#6243=EDGE_CURVE('',#5109,#5108,#2857,.T.);
#6244=EDGE_CURVE('',#5109,#4932,#2858,.T.);
#6245=EDGE_CURVE('',#4934,#5110,#2859,.T.);
#6246=EDGE_CURVE('',#5110,#5111,#2860,.T.);
#6247=EDGE_CURVE('',#4935,#5111,#2861,.T.);
#6248=EDGE_CURVE('',#5110,#5109,#2862,.T.);
#6249=EDGE_CURVE('',#5111,#5108,#2863,.T.);
#6250=EDGE_CURVE('',#5112,#4937,#2864,.T.);
#6251=EDGE_CURVE('',#5113,#5112,#2865,.T.);
#6252=EDGE_CURVE('',#5113,#4936,#2866,.T.);
#6253=EDGE_CURVE('',#4938,#5114,#2867,.T.);
#6254=EDGE_CURVE('',#5114,#5115,#2868,.T.);
#6255=EDGE_CURVE('',#4939,#5115,#2869,.T.);
#6256=EDGE_CURVE('',#5114,#5113,#2870,.T.);
#6257=EDGE_CURVE('',#5115,#5112,#2871,.T.);
#6258=EDGE_CURVE('',#5116,#4941,#2872,.T.);
#6259=EDGE_CURVE('',#5117,#5116,#2873,.T.);
#6260=EDGE_CURVE('',#5117,#4940,#2874,.T.);
#6261=EDGE_CURVE('',#4942,#5118,#2875,.T.);
#6262=EDGE_CURVE('',#5118,#5119,#2876,.T.);
#6263=EDGE_CURVE('',#4943,#5119,#2877,.T.);
#6264=EDGE_CURVE('',#5118,#5117,#2878,.T.);
#6265=EDGE_CURVE('',#5119,#5116,#2879,.T.);
#6266=EDGE_CURVE('',#5120,#4945,#2880,.T.);
#6267=EDGE_CURVE('',#5121,#5120,#2881,.T.);
#6268=EDGE_CURVE('',#5121,#4944,#2882,.T.);
#6269=EDGE_CURVE('',#4946,#5122,#2883,.T.);
#6270=EDGE_CURVE('',#5122,#5123,#2884,.T.);
#6271=EDGE_CURVE('',#4947,#5123,#2885,.T.);
#6272=EDGE_CURVE('',#5122,#5121,#2886,.T.);
#6273=EDGE_CURVE('',#5123,#5120,#2887,.T.);
#6274=EDGE_CURVE('',#5124,#4949,#2888,.T.);
#6275=EDGE_CURVE('',#5125,#5124,#2889,.T.);
#6276=EDGE_CURVE('',#5125,#4948,#2890,.T.);
#6277=EDGE_CURVE('',#4950,#5126,#2891,.T.);
#6278=EDGE_CURVE('',#5126,#5127,#2892,.T.);
#6279=EDGE_CURVE('',#4951,#5127,#2893,.T.);
#6280=EDGE_CURVE('',#5126,#5125,#2894,.T.);
#6281=EDGE_CURVE('',#5127,#5124,#2895,.T.);
#6282=EDGE_CURVE('',#5128,#4953,#2896,.T.);
#6283=EDGE_CURVE('',#5129,#5128,#2897,.T.);
#6284=EDGE_CURVE('',#5129,#4952,#2898,.T.);
#6285=EDGE_CURVE('',#4954,#5130,#2899,.T.);
#6286=EDGE_CURVE('',#5130,#5131,#2900,.T.);
#6287=EDGE_CURVE('',#4955,#5131,#2901,.T.);
#6288=EDGE_CURVE('',#5130,#5129,#2902,.T.);
#6289=EDGE_CURVE('',#5131,#5128,#2903,.T.);
#6290=EDGE_CURVE('',#5132,#4957,#2904,.T.);
#6291=EDGE_CURVE('',#5133,#5132,#2905,.T.);
#6292=EDGE_CURVE('',#5133,#4956,#2906,.T.);
#6293=EDGE_CURVE('',#4958,#5134,#2907,.T.);
#6294=EDGE_CURVE('',#5134,#5135,#2908,.T.);
#6295=EDGE_CURVE('',#4959,#5135,#2909,.T.);
#6296=EDGE_CURVE('',#5134,#5133,#2910,.T.);
#6297=EDGE_CURVE('',#5135,#5132,#2911,.T.);
#6298=EDGE_CURVE('',#5136,#4961,#2912,.T.);
#6299=EDGE_CURVE('',#5137,#5136,#2913,.T.);
#6300=EDGE_CURVE('',#5137,#4960,#2914,.T.);
#6301=EDGE_CURVE('',#4962,#5138,#2915,.T.);
#6302=EDGE_CURVE('',#5138,#5139,#2916,.T.);
#6303=EDGE_CURVE('',#4963,#5139,#2917,.T.);
#6304=EDGE_CURVE('',#5138,#5137,#2918,.T.);
#6305=EDGE_CURVE('',#5139,#5136,#2919,.T.);
#6306=EDGE_CURVE('',#5140,#4965,#2920,.T.);
#6307=EDGE_CURVE('',#5141,#5140,#2921,.T.);
#6308=EDGE_CURVE('',#5141,#4964,#2922,.T.);
#6309=EDGE_CURVE('',#4966,#5142,#2923,.T.);
#6310=EDGE_CURVE('',#5142,#5143,#2924,.T.);
#6311=EDGE_CURVE('',#4967,#5143,#2925,.T.);
#6312=EDGE_CURVE('',#5142,#5141,#2926,.T.);
#6313=EDGE_CURVE('',#5143,#5140,#2927,.T.);
#6314=EDGE_CURVE('',#5144,#4969,#2928,.T.);
#6315=EDGE_CURVE('',#5145,#5144,#2929,.T.);
#6316=EDGE_CURVE('',#5145,#4968,#2930,.T.);
#6317=EDGE_CURVE('',#4970,#5146,#2931,.T.);
#6318=EDGE_CURVE('',#5146,#5147,#2932,.T.);
#6319=EDGE_CURVE('',#4971,#5147,#2933,.T.);
#6320=EDGE_CURVE('',#5146,#5145,#2934,.T.);
#6321=EDGE_CURVE('',#5147,#5144,#2935,.T.);
#6322=EDGE_CURVE('',#5148,#4989,#2936,.T.);
#6323=EDGE_CURVE('',#5149,#5148,#2937,.T.);
#6324=EDGE_CURVE('',#5149,#4988,#2938,.T.);
#6325=EDGE_CURVE('',#4990,#5150,#2939,.T.);
#6326=EDGE_CURVE('',#5150,#5151,#2940,.T.);
#6327=EDGE_CURVE('',#4991,#5151,#2941,.T.);
#6328=EDGE_CURVE('',#5150,#5149,#2942,.T.);
#6329=EDGE_CURVE('',#5151,#5148,#2943,.T.);
#6330=EDGE_CURVE('',#5152,#4993,#2944,.T.);
#6331=EDGE_CURVE('',#5153,#5152,#2945,.T.);
#6332=EDGE_CURVE('',#5153,#4992,#2946,.T.);
#6333=EDGE_CURVE('',#4994,#5154,#2947,.T.);
#6334=EDGE_CURVE('',#5154,#5155,#2948,.T.);
#6335=EDGE_CURVE('',#4995,#5155,#2949,.T.);
#6336=EDGE_CURVE('',#5154,#5153,#2950,.T.);
#6337=EDGE_CURVE('',#5155,#5152,#2951,.T.);
#6338=EDGE_CURVE('',#5156,#4997,#2952,.T.);
#6339=EDGE_CURVE('',#5157,#5156,#2953,.T.);
#6340=EDGE_CURVE('',#5157,#4996,#2954,.T.);
#6341=EDGE_CURVE('',#4998,#5158,#2955,.T.);
#6342=EDGE_CURVE('',#5158,#5159,#2956,.T.);
#6343=EDGE_CURVE('',#4999,#5159,#2957,.T.);
#6344=EDGE_CURVE('',#5158,#5157,#2958,.T.);
#6345=EDGE_CURVE('',#5159,#5156,#2959,.T.);
#6346=EDGE_CURVE('',#5160,#5001,#2960,.T.);
#6347=EDGE_CURVE('',#5161,#5160,#2961,.T.);
#6348=EDGE_CURVE('',#5161,#5000,#2962,.T.);
#6349=EDGE_CURVE('',#5002,#5162,#2963,.T.);
#6350=EDGE_CURVE('',#5162,#5163,#2964,.T.);
#6351=EDGE_CURVE('',#5003,#5163,#2965,.T.);
#6352=EDGE_CURVE('',#5162,#5161,#2966,.T.);
#6353=EDGE_CURVE('',#5163,#5160,#2967,.T.);
#6354=EDGE_CURVE('',#5164,#5005,#2968,.T.);
#6355=EDGE_CURVE('',#5165,#5164,#2969,.T.);
#6356=EDGE_CURVE('',#5165,#5004,#2970,.T.);
#6357=EDGE_CURVE('',#5006,#5166,#2971,.T.);
#6358=EDGE_CURVE('',#5166,#5167,#2972,.T.);
#6359=EDGE_CURVE('',#5007,#5167,#2973,.T.);
#6360=EDGE_CURVE('',#5166,#5165,#2974,.T.);
#6361=EDGE_CURVE('',#5167,#5164,#2975,.T.);
#6362=EDGE_CURVE('',#5168,#5009,#2976,.T.);
#6363=EDGE_CURVE('',#5169,#5168,#2977,.T.);
#6364=EDGE_CURVE('',#5169,#5008,#2978,.T.);
#6365=EDGE_CURVE('',#5010,#5170,#2979,.T.);
#6366=EDGE_CURVE('',#5170,#5171,#2980,.T.);
#6367=EDGE_CURVE('',#5011,#5171,#2981,.T.);
#6368=EDGE_CURVE('',#5170,#5169,#2982,.T.);
#6369=EDGE_CURVE('',#5171,#5168,#2983,.T.);
#6370=EDGE_CURVE('',#5172,#5013,#2984,.T.);
#6371=EDGE_CURVE('',#5173,#5172,#2985,.T.);
#6372=EDGE_CURVE('',#5173,#5012,#2986,.T.);
#6373=EDGE_CURVE('',#5014,#5174,#2987,.T.);
#6374=EDGE_CURVE('',#5174,#5175,#2988,.T.);
#6375=EDGE_CURVE('',#5015,#5175,#2989,.T.);
#6376=EDGE_CURVE('',#5174,#5173,#2990,.T.);
#6377=EDGE_CURVE('',#5175,#5172,#2991,.T.);
#6378=EDGE_CURVE('',#5176,#5017,#2992,.T.);
#6379=EDGE_CURVE('',#5177,#5176,#2993,.T.);
#6380=EDGE_CURVE('',#5177,#5016,#2994,.T.);
#6381=EDGE_CURVE('',#5018,#5178,#2995,.T.);
#6382=EDGE_CURVE('',#5178,#5179,#2996,.T.);
#6383=EDGE_CURVE('',#5019,#5179,#2997,.T.);
#6384=EDGE_CURVE('',#5178,#5177,#2998,.T.);
#6385=EDGE_CURVE('',#5179,#5176,#2999,.T.);
#6386=EDGE_CURVE('',#5180,#5021,#3000,.T.);
#6387=EDGE_CURVE('',#5181,#5180,#3001,.T.);
#6388=EDGE_CURVE('',#5181,#5020,#3002,.T.);
#6389=EDGE_CURVE('',#5022,#5182,#3003,.T.);
#6390=EDGE_CURVE('',#5182,#5183,#3004,.T.);
#6391=EDGE_CURVE('',#5023,#5183,#3005,.T.);
#6392=EDGE_CURVE('',#5182,#5181,#3006,.T.);
#6393=EDGE_CURVE('',#5183,#5180,#3007,.T.);
#6394=EDGE_CURVE('',#5184,#5025,#3008,.T.);
#6395=EDGE_CURVE('',#5185,#5184,#3009,.T.);
#6396=EDGE_CURVE('',#5185,#5024,#3010,.T.);
#6397=EDGE_CURVE('',#5026,#5186,#3011,.T.);
#6398=EDGE_CURVE('',#5186,#5187,#3012,.T.);
#6399=EDGE_CURVE('',#5027,#5187,#3013,.T.);
#6400=EDGE_CURVE('',#5186,#5185,#3014,.T.);
#6401=EDGE_CURVE('',#5187,#5184,#3015,.T.);
#6402=EDGE_CURVE('',#5188,#5029,#3016,.T.);
#6403=EDGE_CURVE('',#5189,#5188,#3017,.T.);
#6404=EDGE_CURVE('',#5189,#5028,#3018,.T.);
#6405=EDGE_CURVE('',#5030,#5190,#3019,.T.);
#6406=EDGE_CURVE('',#5190,#5191,#3020,.T.);
#6407=EDGE_CURVE('',#5031,#5191,#3021,.T.);
#6408=EDGE_CURVE('',#5190,#5189,#3022,.T.);
#6409=EDGE_CURVE('',#5191,#5188,#3023,.T.);
#6410=EDGE_CURVE('',#5192,#5033,#3024,.T.);
#6411=EDGE_CURVE('',#5193,#5192,#3025,.T.);
#6412=EDGE_CURVE('',#5193,#5032,#3026,.T.);
#6413=EDGE_CURVE('',#5034,#5194,#3027,.T.);
#6414=EDGE_CURVE('',#5194,#5195,#3028,.T.);
#6415=EDGE_CURVE('',#5035,#5195,#3029,.T.);
#6416=EDGE_CURVE('',#5194,#5193,#3030,.T.);
#6417=EDGE_CURVE('',#5195,#5192,#3031,.T.);
#6418=EDGE_CURVE('',#5196,#5037,#3032,.T.);
#6419=EDGE_CURVE('',#5197,#5196,#3033,.T.);
#6420=EDGE_CURVE('',#5197,#5036,#3034,.T.);
#6421=EDGE_CURVE('',#5038,#5198,#3035,.T.);
#6422=EDGE_CURVE('',#5198,#5199,#3036,.T.);
#6423=EDGE_CURVE('',#5039,#5199,#3037,.T.);
#6424=EDGE_CURVE('',#5198,#5197,#3038,.T.);
#6425=EDGE_CURVE('',#5199,#5196,#3039,.T.);
#6426=EDGE_CURVE('',#5200,#5041,#3040,.T.);
#6427=EDGE_CURVE('',#5201,#5200,#3041,.T.);
#6428=EDGE_CURVE('',#5201,#5040,#3042,.T.);
#6429=EDGE_CURVE('',#5042,#5202,#3043,.T.);
#6430=EDGE_CURVE('',#5202,#5203,#3044,.T.);
#6431=EDGE_CURVE('',#5043,#5203,#3045,.T.);
#6432=EDGE_CURVE('',#5202,#5201,#3046,.T.);
#6433=EDGE_CURVE('',#5203,#5200,#3047,.T.);
#6434=EDGE_CURVE('',#5204,#5045,#3048,.T.);
#6435=EDGE_CURVE('',#5205,#5204,#3049,.T.);
#6436=EDGE_CURVE('',#5205,#5044,#3050,.T.);
#6437=EDGE_CURVE('',#5046,#5206,#3051,.T.);
#6438=EDGE_CURVE('',#5206,#5207,#3052,.T.);
#6439=EDGE_CURVE('',#5047,#5207,#3053,.T.);
#6440=EDGE_CURVE('',#5206,#5205,#3054,.T.);
#6441=EDGE_CURVE('',#5207,#5204,#3055,.T.);
#7881=ORIENTED_EDGE('',*,*,#5953,.T.);
#7882=ORIENTED_EDGE('',*,*,#5954,.T.);
#7883=ORIENTED_EDGE('',*,*,#5955,.F.);
#7884=ORIENTED_EDGE('',*,*,#5954,.F.);
#7885=ORIENTED_EDGE('',*,*,#5956,.T.);
#7886=ORIENTED_EDGE('',*,*,#5957,.T.);
#7887=ORIENTED_EDGE('',*,*,#5958,.F.);
#7888=ORIENTED_EDGE('',*,*,#5959,.F.);
#7889=ORIENTED_EDGE('',*,*,#5960,.T.);
#7890=ORIENTED_EDGE('',*,*,#5961,.T.);
#7891=ORIENTED_EDGE('',*,*,#5962,.F.);
#7892=ORIENTED_EDGE('',*,*,#5961,.F.);
#7893=ORIENTED_EDGE('',*,*,#5963,.T.);
#7894=ORIENTED_EDGE('',*,*,#5964,.F.);
#7895=ORIENTED_EDGE('',*,*,#5965,.F.);
#7896=ORIENTED_EDGE('',*,*,#5957,.F.);
#7897=ORIENTED_EDGE('',*,*,#5966,.T.);
#7898=ORIENTED_EDGE('',*,*,#5967,.F.);
#7899=ORIENTED_EDGE('',*,*,#5968,.F.);
#7900=ORIENTED_EDGE('',*,*,#5969,.F.);
#7901=ORIENTED_EDGE('',*,*,#5970,.F.);
#7902=ORIENTED_EDGE('',*,*,#5971,.T.);
#7903=ORIENTED_EDGE('',*,*,#5972,.F.);
#7904=ORIENTED_EDGE('',*,*,#5973,.F.);
#7905=ORIENTED_EDGE('',*,*,#5974,.F.);
#7906=ORIENTED_EDGE('',*,*,#5975,.T.);
#7907=ORIENTED_EDGE('',*,*,#5976,.F.);
#7908=ORIENTED_EDGE('',*,*,#5977,.F.);
#7909=ORIENTED_EDGE('',*,*,#5978,.F.);
#7910=ORIENTED_EDGE('',*,*,#5979,.T.);
#7911=ORIENTED_EDGE('',*,*,#5980,.F.);
#7912=ORIENTED_EDGE('',*,*,#5981,.F.);
#7913=ORIENTED_EDGE('',*,*,#5982,.F.);
#7914=ORIENTED_EDGE('',*,*,#5983,.T.);
#7915=ORIENTED_EDGE('',*,*,#5984,.F.);
#7916=ORIENTED_EDGE('',*,*,#5985,.F.);
#7917=ORIENTED_EDGE('',*,*,#5986,.F.);
#7918=ORIENTED_EDGE('',*,*,#5987,.T.);
#7919=ORIENTED_EDGE('',*,*,#5988,.F.);
#7920=ORIENTED_EDGE('',*,*,#5989,.F.);
#7921=ORIENTED_EDGE('',*,*,#5990,.F.);
#7922=ORIENTED_EDGE('',*,*,#5991,.T.);
#7923=ORIENTED_EDGE('',*,*,#5992,.F.);
#7924=ORIENTED_EDGE('',*,*,#5993,.F.);
#7925=ORIENTED_EDGE('',*,*,#5994,.F.);
#7926=ORIENTED_EDGE('',*,*,#5995,.T.);
#7927=ORIENTED_EDGE('',*,*,#5996,.F.);
#7928=ORIENTED_EDGE('',*,*,#5997,.F.);
#7929=ORIENTED_EDGE('',*,*,#5998,.F.);
#7930=ORIENTED_EDGE('',*,*,#5999,.T.);
#7931=ORIENTED_EDGE('',*,*,#6000,.F.);
#7932=ORIENTED_EDGE('',*,*,#6001,.F.);
#7933=ORIENTED_EDGE('',*,*,#6002,.F.);
#7934=ORIENTED_EDGE('',*,*,#6003,.T.);
#7935=ORIENTED_EDGE('',*,*,#6004,.F.);
#7936=ORIENTED_EDGE('',*,*,#6005,.F.);
#7937=ORIENTED_EDGE('',*,*,#6006,.F.);
#7938=ORIENTED_EDGE('',*,*,#6007,.T.);
#7939=ORIENTED_EDGE('',*,*,#6008,.F.);
#7940=ORIENTED_EDGE('',*,*,#6009,.F.);
#7941=ORIENTED_EDGE('',*,*,#6010,.F.);
#7942=ORIENTED_EDGE('',*,*,#6011,.T.);
#7943=ORIENTED_EDGE('',*,*,#6012,.F.);
#7944=ORIENTED_EDGE('',*,*,#6013,.F.);
#7945=ORIENTED_EDGE('',*,*,#6014,.F.);
#7946=ORIENTED_EDGE('',*,*,#6015,.T.);
#7947=ORIENTED_EDGE('',*,*,#6016,.F.);
#7948=ORIENTED_EDGE('',*,*,#6017,.F.);
#7949=ORIENTED_EDGE('',*,*,#6018,.F.);
#7950=ORIENTED_EDGE('',*,*,#6019,.T.);
#7951=ORIENTED_EDGE('',*,*,#6020,.F.);
#7952=ORIENTED_EDGE('',*,*,#6021,.F.);
#7953=ORIENTED_EDGE('',*,*,#6022,.F.);
#7954=ORIENTED_EDGE('',*,*,#6023,.T.);
#7955=ORIENTED_EDGE('',*,*,#6024,.F.);
#7956=ORIENTED_EDGE('',*,*,#6025,.F.);
#7957=ORIENTED_EDGE('',*,*,#6026,.F.);
#7958=ORIENTED_EDGE('',*,*,#6027,.T.);
#7959=ORIENTED_EDGE('',*,*,#6028,.F.);
#7960=ORIENTED_EDGE('',*,*,#6029,.F.);
#7961=ORIENTED_EDGE('',*,*,#6030,.F.);
#7962=ORIENTED_EDGE('',*,*,#6031,.T.);
#7963=ORIENTED_EDGE('',*,*,#6032,.F.);
#7964=ORIENTED_EDGE('',*,*,#6033,.F.);
#7965=ORIENTED_EDGE('',*,*,#6034,.F.);
#7966=ORIENTED_EDGE('',*,*,#6035,.T.);
#7967=ORIENTED_EDGE('',*,*,#6036,.F.);
#7968=ORIENTED_EDGE('',*,*,#6037,.F.);
#7969=ORIENTED_EDGE('',*,*,#6038,.F.);
#7970=ORIENTED_EDGE('',*,*,#6039,.T.);
#7971=ORIENTED_EDGE('',*,*,#6040,.F.);
#7972=ORIENTED_EDGE('',*,*,#6041,.F.);
#7973=ORIENTED_EDGE('',*,*,#6042,.F.);
#7974=ORIENTED_EDGE('',*,*,#6043,.T.);
#7975=ORIENTED_EDGE('',*,*,#6044,.F.);
#7976=ORIENTED_EDGE('',*,*,#6045,.F.);
#7977=ORIENTED_EDGE('',*,*,#6046,.F.);
#7978=ORIENTED_EDGE('',*,*,#6047,.T.);
#7979=ORIENTED_EDGE('',*,*,#6048,.F.);
#7980=ORIENTED_EDGE('',*,*,#6049,.F.);
#7981=ORIENTED_EDGE('',*,*,#6050,.F.);
#7982=ORIENTED_EDGE('',*,*,#6051,.T.);
#7983=ORIENTED_EDGE('',*,*,#6052,.F.);
#7984=ORIENTED_EDGE('',*,*,#6053,.F.);
#7985=ORIENTED_EDGE('',*,*,#6054,.F.);
#7986=ORIENTED_EDGE('',*,*,#6055,.T.);
#7987=ORIENTED_EDGE('',*,*,#6056,.F.);
#7988=ORIENTED_EDGE('',*,*,#6057,.F.);
#7989=ORIENTED_EDGE('',*,*,#6058,.F.);
#7990=ORIENTED_EDGE('',*,*,#6059,.T.);
#7991=ORIENTED_EDGE('',*,*,#6060,.F.);
#7992=ORIENTED_EDGE('',*,*,#6061,.F.);
#7993=ORIENTED_EDGE('',*,*,#6062,.F.);
#7994=ORIENTED_EDGE('',*,*,#6063,.T.);
#7995=ORIENTED_EDGE('',*,*,#6064,.F.);
#7996=ORIENTED_EDGE('',*,*,#6065,.F.);
#7997=ORIENTED_EDGE('',*,*,#6066,.F.);
#7998=ORIENTED_EDGE('',*,*,#6067,.T.);
#7999=ORIENTED_EDGE('',*,*,#6068,.F.);
#8000=ORIENTED_EDGE('',*,*,#6069,.F.);
#8001=ORIENTED_EDGE('',*,*,#6070,.F.);
#8002=ORIENTED_EDGE('',*,*,#6071,.T.);
#8003=ORIENTED_EDGE('',*,*,#6072,.F.);
#8004=ORIENTED_EDGE('',*,*,#6073,.F.);
#8005=ORIENTED_EDGE('',*,*,#6074,.F.);
#8006=ORIENTED_EDGE('',*,*,#6075,.T.);
#8007=ORIENTED_EDGE('',*,*,#6076,.F.);
#8008=ORIENTED_EDGE('',*,*,#6077,.F.);
#8009=ORIENTED_EDGE('',*,*,#6078,.F.);
#8010=ORIENTED_EDGE('',*,*,#6079,.T.);
#8011=ORIENTED_EDGE('',*,*,#6080,.F.);
#8012=ORIENTED_EDGE('',*,*,#6081,.F.);
#8013=ORIENTED_EDGE('',*,*,#6082,.F.);
#8014=ORIENTED_EDGE('',*,*,#6083,.T.);
#8015=ORIENTED_EDGE('',*,*,#6084,.F.);
#8016=ORIENTED_EDGE('',*,*,#6085,.F.);
#8017=ORIENTED_EDGE('',*,*,#6086,.F.);
#8018=ORIENTED_EDGE('',*,*,#6087,.T.);
#8019=ORIENTED_EDGE('',*,*,#6088,.F.);
#8020=ORIENTED_EDGE('',*,*,#6089,.F.);
#8021=ORIENTED_EDGE('',*,*,#6090,.F.);
#8022=ORIENTED_EDGE('',*,*,#6091,.T.);
#8023=ORIENTED_EDGE('',*,*,#6092,.F.);
#8024=ORIENTED_EDGE('',*,*,#6093,.F.);
#8025=ORIENTED_EDGE('',*,*,#6094,.F.);
#8026=ORIENTED_EDGE('',*,*,#6095,.T.);
#8027=ORIENTED_EDGE('',*,*,#6096,.F.);
#8028=ORIENTED_EDGE('',*,*,#6097,.F.);
#8029=ORIENTED_EDGE('',*,*,#6098,.F.);
#8030=ORIENTED_EDGE('',*,*,#6099,.T.);
#8031=ORIENTED_EDGE('',*,*,#6100,.F.);
#8032=ORIENTED_EDGE('',*,*,#6101,.F.);
#8033=ORIENTED_EDGE('',*,*,#6102,.F.);
#8034=ORIENTED_EDGE('',*,*,#6103,.T.);
#8035=ORIENTED_EDGE('',*,*,#6104,.F.);
#8036=ORIENTED_EDGE('',*,*,#6105,.F.);
#8037=ORIENTED_EDGE('',*,*,#6106,.F.);
#8038=ORIENTED_EDGE('',*,*,#6107,.T.);
#8039=ORIENTED_EDGE('',*,*,#6108,.F.);
#8040=ORIENTED_EDGE('',*,*,#6109,.F.);
#8041=ORIENTED_EDGE('',*,*,#6110,.F.);
#8042=ORIENTED_EDGE('',*,*,#6111,.T.);
#8043=ORIENTED_EDGE('',*,*,#6112,.F.);
#8044=ORIENTED_EDGE('',*,*,#6113,.F.);
#8045=ORIENTED_EDGE('',*,*,#6114,.F.);
#8046=ORIENTED_EDGE('',*,*,#6115,.T.);
#8047=ORIENTED_EDGE('',*,*,#6116,.F.);
#8048=ORIENTED_EDGE('',*,*,#6117,.F.);
#8049=ORIENTED_EDGE('',*,*,#6118,.F.);
#8050=ORIENTED_EDGE('',*,*,#6119,.T.);
#8051=ORIENTED_EDGE('',*,*,#6120,.F.);
#8052=ORIENTED_EDGE('',*,*,#6121,.F.);
#8053=ORIENTED_EDGE('',*,*,#5962,.T.);
#8054=ORIENTED_EDGE('',*,*,#5953,.F.);
#8055=ORIENTED_EDGE('',*,*,#5956,.F.);
#8056=ORIENTED_EDGE('',*,*,#5955,.T.);
#8057=ORIENTED_EDGE('',*,*,#5970,.T.);
#8058=ORIENTED_EDGE('',*,*,#6122,.F.);
#8059=ORIENTED_EDGE('',*,*,#6123,.F.);
#8060=ORIENTED_EDGE('',*,*,#6124,.T.);
#8061=ORIENTED_EDGE('',*,*,#5972,.T.);
#8062=ORIENTED_EDGE('',*,*,#6125,.T.);
#8063=ORIENTED_EDGE('',*,*,#6126,.T.);
#8064=ORIENTED_EDGE('',*,*,#6127,.F.);
#8065=ORIENTED_EDGE('',*,*,#6124,.F.);
#8066=ORIENTED_EDGE('',*,*,#6128,.F.);
#8067=ORIENTED_EDGE('',*,*,#6125,.F.);
#8068=ORIENTED_EDGE('',*,*,#5971,.F.);
#8069=ORIENTED_EDGE('',*,*,#5973,.T.);
#8070=ORIENTED_EDGE('',*,*,#6127,.T.);
#8071=ORIENTED_EDGE('',*,*,#6129,.T.);
#8072=ORIENTED_EDGE('',*,*,#6122,.T.);
#8073=ORIENTED_EDGE('',*,*,#6129,.F.);
#8074=ORIENTED_EDGE('',*,*,#6126,.F.);
#8075=ORIENTED_EDGE('',*,*,#6128,.T.);
#8076=ORIENTED_EDGE('',*,*,#6123,.T.);
#8077=ORIENTED_EDGE('',*,*,#5974,.T.);
#8078=ORIENTED_EDGE('',*,*,#6130,.F.);
#8079=ORIENTED_EDGE('',*,*,#6131,.F.);
#8080=ORIENTED_EDGE('',*,*,#6132,.T.);
#8081=ORIENTED_EDGE('',*,*,#5976,.T.);
#8082=ORIENTED_EDGE('',*,*,#6133,.T.);
#8083=ORIENTED_EDGE('',*,*,#6134,.T.);
#8084=ORIENTED_EDGE('',*,*,#6135,.F.);
#8085=ORIENTED_EDGE('',*,*,#6132,.F.);
#8086=ORIENTED_EDGE('',*,*,#6136,.F.);
#8087=ORIENTED_EDGE('',*,*,#6133,.F.);
#8088=ORIENTED_EDGE('',*,*,#5975,.F.);
#8089=ORIENTED_EDGE('',*,*,#5977,.T.);
#8090=ORIENTED_EDGE('',*,*,#6135,.T.);
#8091=ORIENTED_EDGE('',*,*,#6137,.T.);
#8092=ORIENTED_EDGE('',*,*,#6130,.T.);
#8093=ORIENTED_EDGE('',*,*,#6137,.F.);
#8094=ORIENTED_EDGE('',*,*,#6134,.F.);
#8095=ORIENTED_EDGE('',*,*,#6136,.T.);
#8096=ORIENTED_EDGE('',*,*,#6131,.T.);
#8097=ORIENTED_EDGE('',*,*,#5978,.T.);
#8098=ORIENTED_EDGE('',*,*,#6138,.F.);
#8099=ORIENTED_EDGE('',*,*,#6139,.F.);
#8100=ORIENTED_EDGE('',*,*,#6140,.T.);
#8101=ORIENTED_EDGE('',*,*,#5980,.T.);
#8102=ORIENTED_EDGE('',*,*,#6141,.T.);
#8103=ORIENTED_EDGE('',*,*,#6142,.T.);
#8104=ORIENTED_EDGE('',*,*,#6143,.F.);
#8105=ORIENTED_EDGE('',*,*,#6140,.F.);
#8106=ORIENTED_EDGE('',*,*,#6144,.F.);
#8107=ORIENTED_EDGE('',*,*,#6141,.F.);
#8108=ORIENTED_EDGE('',*,*,#5979,.F.);
#8109=ORIENTED_EDGE('',*,*,#5981,.T.);
#8110=ORIENTED_EDGE('',*,*,#6143,.T.);
#8111=ORIENTED_EDGE('',*,*,#6145,.T.);
#8112=ORIENTED_EDGE('',*,*,#6138,.T.);
#8113=ORIENTED_EDGE('',*,*,#6145,.F.);
#8114=ORIENTED_EDGE('',*,*,#6142,.F.);
#8115=ORIENTED_EDGE('',*,*,#6144,.T.);
#8116=ORIENTED_EDGE('',*,*,#6139,.T.);
#8117=ORIENTED_EDGE('',*,*,#5969,.T.);
#8118=ORIENTED_EDGE('',*,*,#6146,.F.);
#8119=ORIENTED_EDGE('',*,*,#6147,.F.);
#8120=ORIENTED_EDGE('',*,*,#6148,.T.);
#8121=ORIENTED_EDGE('',*,*,#5967,.T.);
#8122=ORIENTED_EDGE('',*,*,#6149,.T.);
#8123=ORIENTED_EDGE('',*,*,#6150,.T.);
#8124=ORIENTED_EDGE('',*,*,#6151,.F.);
#8125=ORIENTED_EDGE('',*,*,#6148,.F.);
#8126=ORIENTED_EDGE('',*,*,#6152,.F.);
#8127=ORIENTED_EDGE('',*,*,#6149,.F.);
#8128=ORIENTED_EDGE('',*,*,#5966,.F.);
#8129=ORIENTED_EDGE('',*,*,#5968,.T.);
#8130=ORIENTED_EDGE('',*,*,#6151,.T.);
#8131=ORIENTED_EDGE('',*,*,#6153,.T.);
#8132=ORIENTED_EDGE('',*,*,#6146,.T.);
#8133=ORIENTED_EDGE('',*,*,#6153,.F.);
#8134=ORIENTED_EDGE('',*,*,#6150,.F.);
#8135=ORIENTED_EDGE('',*,*,#6152,.T.);
#8136=ORIENTED_EDGE('',*,*,#6147,.T.);
#8137=ORIENTED_EDGE('',*,*,#6046,.T.);
#8138=ORIENTED_EDGE('',*,*,#6154,.F.);
#8139=ORIENTED_EDGE('',*,*,#6155,.F.);
#8140=ORIENTED_EDGE('',*,*,#6156,.T.);
#8141=ORIENTED_EDGE('',*,*,#6048,.T.);
#8142=ORIENTED_EDGE('',*,*,#6157,.T.);
#8143=ORIENTED_EDGE('',*,*,#6158,.T.);
#8144=ORIENTED_EDGE('',*,*,#6159,.F.);
#8145=ORIENTED_EDGE('',*,*,#6156,.F.);
#8146=ORIENTED_EDGE('',*,*,#6160,.F.);
#8147=ORIENTED_EDGE('',*,*,#6157,.F.);
#8148=ORIENTED_EDGE('',*,*,#6047,.F.);
#8149=ORIENTED_EDGE('',*,*,#6049,.T.);
#8150=ORIENTED_EDGE('',*,*,#6159,.T.);
#8151=ORIENTED_EDGE('',*,*,#6161,.T.);
#8152=ORIENTED_EDGE('',*,*,#6154,.T.);
#8153=ORIENTED_EDGE('',*,*,#6161,.F.);
#8154=ORIENTED_EDGE('',*,*,#6158,.F.);
#8155=ORIENTED_EDGE('',*,*,#6160,.T.);
#8156=ORIENTED_EDGE('',*,*,#6155,.T.);
#8157=ORIENTED_EDGE('',*,*,#6050,.T.);
#8158=ORIENTED_EDGE('',*,*,#6162,.F.);
#8159=ORIENTED_EDGE('',*,*,#6163,.F.);
#8160=ORIENTED_EDGE('',*,*,#6164,.T.);
#8161=ORIENTED_EDGE('',*,*,#6052,.T.);
#8162=ORIENTED_EDGE('',*,*,#6165,.T.);
#8163=ORIENTED_EDGE('',*,*,#6166,.T.);
#8164=ORIENTED_EDGE('',*,*,#6167,.F.);
#8165=ORIENTED_EDGE('',*,*,#6164,.F.);
#8166=ORIENTED_EDGE('',*,*,#6168,.F.);
#8167=ORIENTED_EDGE('',*,*,#6165,.F.);
#8168=ORIENTED_EDGE('',*,*,#6051,.F.);
#8169=ORIENTED_EDGE('',*,*,#6053,.T.);
#8170=ORIENTED_EDGE('',*,*,#6167,.T.);
#8171=ORIENTED_EDGE('',*,*,#6169,.T.);
#8172=ORIENTED_EDGE('',*,*,#6162,.T.);
#8173=ORIENTED_EDGE('',*,*,#6169,.F.);
#8174=ORIENTED_EDGE('',*,*,#6166,.F.);
#8175=ORIENTED_EDGE('',*,*,#6168,.T.);
#8176=ORIENTED_EDGE('',*,*,#6163,.T.);
#8177=ORIENTED_EDGE('',*,*,#6054,.T.);
#8178=ORIENTED_EDGE('',*,*,#6170,.F.);
#8179=ORIENTED_EDGE('',*,*,#6171,.F.);
#8180=ORIENTED_EDGE('',*,*,#6172,.T.);
#8181=ORIENTED_EDGE('',*,*,#6056,.T.);
#8182=ORIENTED_EDGE('',*,*,#6173,.T.);
#8183=ORIENTED_EDGE('',*,*,#6174,.T.);
#8184=ORIENTED_EDGE('',*,*,#6175,.F.);
#8185=ORIENTED_EDGE('',*,*,#6172,.F.);
#8186=ORIENTED_EDGE('',*,*,#6176,.F.);
#8187=ORIENTED_EDGE('',*,*,#6173,.F.);
#8188=ORIENTED_EDGE('',*,*,#6055,.F.);
#8189=ORIENTED_EDGE('',*,*,#6057,.T.);
#8190=ORIENTED_EDGE('',*,*,#6175,.T.);
#8191=ORIENTED_EDGE('',*,*,#6177,.T.);
#8192=ORIENTED_EDGE('',*,*,#6170,.T.);
#8193=ORIENTED_EDGE('',*,*,#6177,.F.);
#8194=ORIENTED_EDGE('',*,*,#6174,.F.);
#8195=ORIENTED_EDGE('',*,*,#6176,.T.);
#8196=ORIENTED_EDGE('',*,*,#6171,.T.);
#8197=ORIENTED_EDGE('',*,*,#5959,.T.);
#8198=ORIENTED_EDGE('',*,*,#6178,.F.);
#8199=ORIENTED_EDGE('',*,*,#6179,.F.);
#8200=ORIENTED_EDGE('',*,*,#6180,.T.);
#8201=ORIENTED_EDGE('',*,*,#5964,.T.);
#8202=ORIENTED_EDGE('',*,*,#6181,.T.);
#8203=ORIENTED_EDGE('',*,*,#6182,.T.);
#8204=ORIENTED_EDGE('',*,*,#6183,.F.);
#8205=ORIENTED_EDGE('',*,*,#6180,.F.);
#8206=ORIENTED_EDGE('',*,*,#6184,.F.);
#8207=ORIENTED_EDGE('',*,*,#6181,.F.);
#8208=ORIENTED_EDGE('',*,*,#5963,.F.);
#8209=ORIENTED_EDGE('',*,*,#5960,.F.);
#8210=ORIENTED_EDGE('',*,*,#5958,.T.);
#8211=ORIENTED_EDGE('',*,*,#5965,.T.);
#8212=ORIENTED_EDGE('',*,*,#6183,.T.);
#8213=ORIENTED_EDGE('',*,*,#6185,.T.);
#8214=ORIENTED_EDGE('',*,*,#6178,.T.);
#8215=ORIENTED_EDGE('',*,*,#6185,.F.);
#8216=ORIENTED_EDGE('',*,*,#6182,.F.);
#8217=ORIENTED_EDGE('',*,*,#6184,.T.);
#8218=ORIENTED_EDGE('',*,*,#6179,.T.);
#8219=ORIENTED_EDGE('',*,*,#6058,.T.);
#8220=ORIENTED_EDGE('',*,*,#6186,.F.);
#8221=ORIENTED_EDGE('',*,*,#6187,.F.);
#8222=ORIENTED_EDGE('',*,*,#6188,.T.);
#8223=ORIENTED_EDGE('',*,*,#6060,.T.);
#8224=ORIENTED_EDGE('',*,*,#6189,.T.);
#8225=ORIENTED_EDGE('',*,*,#6190,.T.);
#8226=ORIENTED_EDGE('',*,*,#6191,.F.);
#8227=ORIENTED_EDGE('',*,*,#6188,.F.);
#8228=ORIENTED_EDGE('',*,*,#6192,.F.);
#8229=ORIENTED_EDGE('',*,*,#6189,.F.);
#8230=ORIENTED_EDGE('',*,*,#6059,.F.);
#8231=ORIENTED_EDGE('',*,*,#6061,.T.);
#8232=ORIENTED_EDGE('',*,*,#6191,.T.);
#8233=ORIENTED_EDGE('',*,*,#6193,.T.);
#8234=ORIENTED_EDGE('',*,*,#6186,.T.);
#8235=ORIENTED_EDGE('',*,*,#6193,.F.);
#8236=ORIENTED_EDGE('',*,*,#6190,.F.);
#8237=ORIENTED_EDGE('',*,*,#6192,.T.);
#8238=ORIENTED_EDGE('',*,*,#6187,.T.);
#8239=ORIENTED_EDGE('',*,*,#5982,.T.);
#8240=ORIENTED_EDGE('',*,*,#6194,.F.);
#8241=ORIENTED_EDGE('',*,*,#6195,.F.);
#8242=ORIENTED_EDGE('',*,*,#6196,.T.);
#8243=ORIENTED_EDGE('',*,*,#5984,.T.);
#8244=ORIENTED_EDGE('',*,*,#6197,.T.);
#8245=ORIENTED_EDGE('',*,*,#6198,.T.);
#8246=ORIENTED_EDGE('',*,*,#6199,.F.);
#8247=ORIENTED_EDGE('',*,*,#6196,.F.);
#8248=ORIENTED_EDGE('',*,*,#6200,.F.);
#8249=ORIENTED_EDGE('',*,*,#6197,.F.);
#8250=ORIENTED_EDGE('',*,*,#5983,.F.);
#8251=ORIENTED_EDGE('',*,*,#5985,.T.);
#8252=ORIENTED_EDGE('',*,*,#6199,.T.);
#8253=ORIENTED_EDGE('',*,*,#6201,.T.);
#8254=ORIENTED_EDGE('',*,*,#6194,.T.);
#8255=ORIENTED_EDGE('',*,*,#6201,.F.);
#8256=ORIENTED_EDGE('',*,*,#6198,.F.);
#8257=ORIENTED_EDGE('',*,*,#6200,.T.);
#8258=ORIENTED_EDGE('',*,*,#6195,.T.);
#8259=ORIENTED_EDGE('',*,*,#5986,.T.);
#8260=ORIENTED_EDGE('',*,*,#6202,.F.);
#8261=ORIENTED_EDGE('',*,*,#6203,.F.);
#8262=ORIENTED_EDGE('',*,*,#6204,.T.);
#8263=ORIENTED_EDGE('',*,*,#5988,.T.);
#8264=ORIENTED_EDGE('',*,*,#6205,.T.);
#8265=ORIENTED_EDGE('',*,*,#6206,.T.);
#8266=ORIENTED_EDGE('',*,*,#6207,.F.);
#8267=ORIENTED_EDGE('',*,*,#6204,.F.);
#8268=ORIENTED_EDGE('',*,*,#6208,.F.);
#8269=ORIENTED_EDGE('',*,*,#6205,.F.);
#8270=ORIENTED_EDGE('',*,*,#5987,.F.);
#8271=ORIENTED_EDGE('',*,*,#5989,.T.);
#8272=ORIENTED_EDGE('',*,*,#6207,.T.);
#8273=ORIENTED_EDGE('',*,*,#6209,.T.);
#8274=ORIENTED_EDGE('',*,*,#6202,.T.);
#8275=ORIENTED_EDGE('',*,*,#6209,.F.);
#8276=ORIENTED_EDGE('',*,*,#6206,.F.);
#8277=ORIENTED_EDGE('',*,*,#6208,.T.);
#8278=ORIENTED_EDGE('',*,*,#6203,.T.);
#8279=ORIENTED_EDGE('',*,*,#5990,.T.);
#8280=ORIENTED_EDGE('',*,*,#6210,.F.);
#8281=ORIENTED_EDGE('',*,*,#6211,.F.);
#8282=ORIENTED_EDGE('',*,*,#6212,.T.);
#8283=ORIENTED_EDGE('',*,*,#5992,.T.);
#8284=ORIENTED_EDGE('',*,*,#6213,.T.);
#8285=ORIENTED_EDGE('',*,*,#6214,.T.);
#8286=ORIENTED_EDGE('',*,*,#6215,.F.);
#8287=ORIENTED_EDGE('',*,*,#6212,.F.);
#8288=ORIENTED_EDGE('',*,*,#6216,.F.);
#8289=ORIENTED_EDGE('',*,*,#6213,.F.);
#8290=ORIENTED_EDGE('',*,*,#5991,.F.);
#8291=ORIENTED_EDGE('',*,*,#5993,.T.);
#8292=ORIENTED_EDGE('',*,*,#6215,.T.);
#8293=ORIENTED_EDGE('',*,*,#6217,.T.);
#8294=ORIENTED_EDGE('',*,*,#6210,.T.);
#8295=ORIENTED_EDGE('',*,*,#6217,.F.);
#8296=ORIENTED_EDGE('',*,*,#6214,.F.);
#8297=ORIENTED_EDGE('',*,*,#6216,.T.);
#8298=ORIENTED_EDGE('',*,*,#6211,.T.);
#8299=ORIENTED_EDGE('',*,*,#5994,.T.);
#8300=ORIENTED_EDGE('',*,*,#6218,.F.);
#8301=ORIENTED_EDGE('',*,*,#6219,.F.);
#8302=ORIENTED_EDGE('',*,*,#6220,.T.);
#8303=ORIENTED_EDGE('',*,*,#5996,.T.);
#8304=ORIENTED_EDGE('',*,*,#6221,.T.);
#8305=ORIENTED_EDGE('',*,*,#6222,.T.);
#8306=ORIENTED_EDGE('',*,*,#6223,.F.);
#8307=ORIENTED_EDGE('',*,*,#6220,.F.);
#8308=ORIENTED_EDGE('',*,*,#6224,.F.);
#8309=ORIENTED_EDGE('',*,*,#6221,.F.);
#8310=ORIENTED_EDGE('',*,*,#5995,.F.);
#8311=ORIENTED_EDGE('',*,*,#5997,.T.);
#8312=ORIENTED_EDGE('',*,*,#6223,.T.);
#8313=ORIENTED_EDGE('',*,*,#6225,.T.);
#8314=ORIENTED_EDGE('',*,*,#6218,.T.);
#8315=ORIENTED_EDGE('',*,*,#6225,.F.);
#8316=ORIENTED_EDGE('',*,*,#6222,.F.);
#8317=ORIENTED_EDGE('',*,*,#6224,.T.);
#8318=ORIENTED_EDGE('',*,*,#6219,.T.);
#8319=ORIENTED_EDGE('',*,*,#5998,.T.);
#8320=ORIENTED_EDGE('',*,*,#6226,.F.);
#8321=ORIENTED_EDGE('',*,*,#6227,.F.);
#8322=ORIENTED_EDGE('',*,*,#6228,.T.);
#8323=ORIENTED_EDGE('',*,*,#6000,.T.);
#8324=ORIENTED_EDGE('',*,*,#6229,.T.);
#8325=ORIENTED_EDGE('',*,*,#6230,.T.);
#8326=ORIENTED_EDGE('',*,*,#6231,.F.);
#8327=ORIENTED_EDGE('',*,*,#6228,.F.);
#8328=ORIENTED_EDGE('',*,*,#6232,.F.);
#8329=ORIENTED_EDGE('',*,*,#6229,.F.);
#8330=ORIENTED_EDGE('',*,*,#5999,.F.);
#8331=ORIENTED_EDGE('',*,*,#6001,.T.);
#8332=ORIENTED_EDGE('',*,*,#6231,.T.);
#8333=ORIENTED_EDGE('',*,*,#6233,.T.);
#8334=ORIENTED_EDGE('',*,*,#6226,.T.);
#8335=ORIENTED_EDGE('',*,*,#6233,.F.);
#8336=ORIENTED_EDGE('',*,*,#6230,.F.);
#8337=ORIENTED_EDGE('',*,*,#6232,.T.);
#8338=ORIENTED_EDGE('',*,*,#6227,.T.);
#8339=ORIENTED_EDGE('',*,*,#6002,.T.);
#8340=ORIENTED_EDGE('',*,*,#6234,.F.);
#8341=ORIENTED_EDGE('',*,*,#6235,.F.);
#8342=ORIENTED_EDGE('',*,*,#6236,.T.);
#8343=ORIENTED_EDGE('',*,*,#6004,.T.);
#8344=ORIENTED_EDGE('',*,*,#6237,.T.);
#8345=ORIENTED_EDGE('',*,*,#6238,.T.);
#8346=ORIENTED_EDGE('',*,*,#6239,.F.);
#8347=ORIENTED_EDGE('',*,*,#6236,.F.);
#8348=ORIENTED_EDGE('',*,*,#6240,.F.);
#8349=ORIENTED_EDGE('',*,*,#6237,.F.);
#8350=ORIENTED_EDGE('',*,*,#6003,.F.);
#8351=ORIENTED_EDGE('',*,*,#6005,.T.);
#8352=ORIENTED_EDGE('',*,*,#6239,.T.);
#8353=ORIENTED_EDGE('',*,*,#6241,.T.);
#8354=ORIENTED_EDGE('',*,*,#6234,.T.);
#8355=ORIENTED_EDGE('',*,*,#6241,.F.);
#8356=ORIENTED_EDGE('',*,*,#6238,.F.);
#8357=ORIENTED_EDGE('',*,*,#6240,.T.);
#8358=ORIENTED_EDGE('',*,*,#6235,.T.);
#8359=ORIENTED_EDGE('',*,*,#6006,.T.);
#8360=ORIENTED_EDGE('',*,*,#6242,.F.);
#8361=ORIENTED_EDGE('',*,*,#6243,.F.);
#8362=ORIENTED_EDGE('',*,*,#6244,.T.);
#8363=ORIENTED_EDGE('',*,*,#6008,.T.);
#8364=ORIENTED_EDGE('',*,*,#6245,.T.);
#8365=ORIENTED_EDGE('',*,*,#6246,.T.);
#8366=ORIENTED_EDGE('',*,*,#6247,.F.);
#8367=ORIENTED_EDGE('',*,*,#6244,.F.);
#8368=ORIENTED_EDGE('',*,*,#6248,.F.);
#8369=ORIENTED_EDGE('',*,*,#6245,.F.);
#8370=ORIENTED_EDGE('',*,*,#6007,.F.);
#8371=ORIENTED_EDGE('',*,*,#6009,.T.);
#8372=ORIENTED_EDGE('',*,*,#6247,.T.);
#8373=ORIENTED_EDGE('',*,*,#6249,.T.);
#8374=ORIENTED_EDGE('',*,*,#6242,.T.);
#8375=ORIENTED_EDGE('',*,*,#6249,.F.);
#8376=ORIENTED_EDGE('',*,*,#6246,.F.);
#8377=ORIENTED_EDGE('',*,*,#6248,.T.);
#8378=ORIENTED_EDGE('',*,*,#6243,.T.);
#8379=ORIENTED_EDGE('',*,*,#6010,.T.);
#8380=ORIENTED_EDGE('',*,*,#6250,.F.);
#8381=ORIENTED_EDGE('',*,*,#6251,.F.);
#8382=ORIENTED_EDGE('',*,*,#6252,.T.);
#8383=ORIENTED_EDGE('',*,*,#6012,.T.);
#8384=ORIENTED_EDGE('',*,*,#6253,.T.);
#8385=ORIENTED_EDGE('',*,*,#6254,.T.);
#8386=ORIENTED_EDGE('',*,*,#6255,.F.);
#8387=ORIENTED_EDGE('',*,*,#6252,.F.);
#8388=ORIENTED_EDGE('',*,*,#6256,.F.);
#8389=ORIENTED_EDGE('',*,*,#6253,.F.);
#8390=ORIENTED_EDGE('',*,*,#6011,.F.);
#8391=ORIENTED_EDGE('',*,*,#6013,.T.);
#8392=ORIENTED_EDGE('',*,*,#6255,.T.);
#8393=ORIENTED_EDGE('',*,*,#6257,.T.);
#8394=ORIENTED_EDGE('',*,*,#6250,.T.);
#8395=ORIENTED_EDGE('',*,*,#6257,.F.);
#8396=ORIENTED_EDGE('',*,*,#6254,.F.);
#8397=ORIENTED_EDGE('',*,*,#6256,.T.);
#8398=ORIENTED_EDGE('',*,*,#6251,.T.);
#8399=ORIENTED_EDGE('',*,*,#6014,.T.);
#8400=ORIENTED_EDGE('',*,*,#6258,.F.);
#8401=ORIENTED_EDGE('',*,*,#6259,.F.);
#8402=ORIENTED_EDGE('',*,*,#6260,.T.);
#8403=ORIENTED_EDGE('',*,*,#6016,.T.);
#8404=ORIENTED_EDGE('',*,*,#6261,.T.);
#8405=ORIENTED_EDGE('',*,*,#6262,.T.);
#8406=ORIENTED_EDGE('',*,*,#6263,.F.);
#8407=ORIENTED_EDGE('',*,*,#6260,.F.);
#8408=ORIENTED_EDGE('',*,*,#6264,.F.);
#8409=ORIENTED_EDGE('',*,*,#6261,.F.);
#8410=ORIENTED_EDGE('',*,*,#6015,.F.);
#8411=ORIENTED_EDGE('',*,*,#6017,.T.);
#8412=ORIENTED_EDGE('',*,*,#6263,.T.);
#8413=ORIENTED_EDGE('',*,*,#6265,.T.);
#8414=ORIENTED_EDGE('',*,*,#6258,.T.);
#8415=ORIENTED_EDGE('',*,*,#6265,.F.);
#8416=ORIENTED_EDGE('',*,*,#6262,.F.);
#8417=ORIENTED_EDGE('',*,*,#6264,.T.);
#8418=ORIENTED_EDGE('',*,*,#6259,.T.);
#8419=ORIENTED_EDGE('',*,*,#6018,.T.);
#8420=ORIENTED_EDGE('',*,*,#6266,.F.);
#8421=ORIENTED_EDGE('',*,*,#6267,.F.);
#8422=ORIENTED_EDGE('',*,*,#6268,.T.);
#8423=ORIENTED_EDGE('',*,*,#6020,.T.);
#8424=ORIENTED_EDGE('',*,*,#6269,.T.);
#8425=ORIENTED_EDGE('',*,*,#6270,.T.);
#8426=ORIENTED_EDGE('',*,*,#6271,.F.);
#8427=ORIENTED_EDGE('',*,*,#6268,.F.);
#8428=ORIENTED_EDGE('',*,*,#6272,.F.);
#8429=ORIENTED_EDGE('',*,*,#6269,.F.);
#8430=ORIENTED_EDGE('',*,*,#6019,.F.);
#8431=ORIENTED_EDGE('',*,*,#6021,.T.);
#8432=ORIENTED_EDGE('',*,*,#6271,.T.);
#8433=ORIENTED_EDGE('',*,*,#6273,.T.);
#8434=ORIENTED_EDGE('',*,*,#6266,.T.);
#8435=ORIENTED_EDGE('',*,*,#6273,.F.);
#8436=ORIENTED_EDGE('',*,*,#6270,.F.);
#8437=ORIENTED_EDGE('',*,*,#6272,.T.);
#8438=ORIENTED_EDGE('',*,*,#6267,.T.);
#8439=ORIENTED_EDGE('',*,*,#6022,.T.);
#8440=ORIENTED_EDGE('',*,*,#6274,.F.);
#8441=ORIENTED_EDGE('',*,*,#6275,.F.);
#8442=ORIENTED_EDGE('',*,*,#6276,.T.);
#8443=ORIENTED_EDGE('',*,*,#6024,.T.);
#8444=ORIENTED_EDGE('',*,*,#6277,.T.);
#8445=ORIENTED_EDGE('',*,*,#6278,.T.);
#8446=ORIENTED_EDGE('',*,*,#6279,.F.);
#8447=ORIENTED_EDGE('',*,*,#6276,.F.);
#8448=ORIENTED_EDGE('',*,*,#6280,.F.);
#8449=ORIENTED_EDGE('',*,*,#6277,.F.);
#8450=ORIENTED_EDGE('',*,*,#6023,.F.);
#8451=ORIENTED_EDGE('',*,*,#6025,.T.);
#8452=ORIENTED_EDGE('',*,*,#6279,.T.);
#8453=ORIENTED_EDGE('',*,*,#6281,.T.);
#8454=ORIENTED_EDGE('',*,*,#6274,.T.);
#8455=ORIENTED_EDGE('',*,*,#6281,.F.);
#8456=ORIENTED_EDGE('',*,*,#6278,.F.);
#8457=ORIENTED_EDGE('',*,*,#6280,.T.);
#8458=ORIENTED_EDGE('',*,*,#6275,.T.);
#8459=ORIENTED_EDGE('',*,*,#6026,.T.);
#8460=ORIENTED_EDGE('',*,*,#6282,.F.);
#8461=ORIENTED_EDGE('',*,*,#6283,.F.);
#8462=ORIENTED_EDGE('',*,*,#6284,.T.);
#8463=ORIENTED_EDGE('',*,*,#6028,.T.);
#8464=ORIENTED_EDGE('',*,*,#6285,.T.);
#8465=ORIENTED_EDGE('',*,*,#6286,.T.);
#8466=ORIENTED_EDGE('',*,*,#6287,.F.);
#8467=ORIENTED_EDGE('',*,*,#6284,.F.);
#8468=ORIENTED_EDGE('',*,*,#6288,.F.);
#8469=ORIENTED_EDGE('',*,*,#6285,.F.);
#8470=ORIENTED_EDGE('',*,*,#6027,.F.);
#8471=ORIENTED_EDGE('',*,*,#6029,.T.);
#8472=ORIENTED_EDGE('',*,*,#6287,.T.);
#8473=ORIENTED_EDGE('',*,*,#6289,.T.);
#8474=ORIENTED_EDGE('',*,*,#6282,.T.);
#8475=ORIENTED_EDGE('',*,*,#6289,.F.);
#8476=ORIENTED_EDGE('',*,*,#6286,.F.);
#8477=ORIENTED_EDGE('',*,*,#6288,.T.);
#8478=ORIENTED_EDGE('',*,*,#6283,.T.);
#8479=ORIENTED_EDGE('',*,*,#6030,.T.);
#8480=ORIENTED_EDGE('',*,*,#6290,.F.);
#8481=ORIENTED_EDGE('',*,*,#6291,.F.);
#8482=ORIENTED_EDGE('',*,*,#6292,.T.);
#8483=ORIENTED_EDGE('',*,*,#6032,.T.);
#8484=ORIENTED_EDGE('',*,*,#6293,.T.);
#8485=ORIENTED_EDGE('',*,*,#6294,.T.);
#8486=ORIENTED_EDGE('',*,*,#6295,.F.);
#8487=ORIENTED_EDGE('',*,*,#6292,.F.);
#8488=ORIENTED_EDGE('',*,*,#6296,.F.);
#8489=ORIENTED_EDGE('',*,*,#6293,.F.);
#8490=ORIENTED_EDGE('',*,*,#6031,.F.);
#8491=ORIENTED_EDGE('',*,*,#6033,.T.);
#8492=ORIENTED_EDGE('',*,*,#6295,.T.);
#8493=ORIENTED_EDGE('',*,*,#6297,.T.);
#8494=ORIENTED_EDGE('',*,*,#6290,.T.);
#8495=ORIENTED_EDGE('',*,*,#6297,.F.);
#8496=ORIENTED_EDGE('',*,*,#6294,.F.);
#8497=ORIENTED_EDGE('',*,*,#6296,.T.);
#8498=ORIENTED_EDGE('',*,*,#6291,.T.);
#8499=ORIENTED_EDGE('',*,*,#6034,.T.);
#8500=ORIENTED_EDGE('',*,*,#6298,.F.);
#8501=ORIENTED_EDGE('',*,*,#6299,.F.);
#8502=ORIENTED_EDGE('',*,*,#6300,.T.);
#8503=ORIENTED_EDGE('',*,*,#6036,.T.);
#8504=ORIENTED_EDGE('',*,*,#6301,.T.);
#8505=ORIENTED_EDGE('',*,*,#6302,.T.);
#8506=ORIENTED_EDGE('',*,*,#6303,.F.);
#8507=ORIENTED_EDGE('',*,*,#6300,.F.);
#8508=ORIENTED_EDGE('',*,*,#6304,.F.);
#8509=ORIENTED_EDGE('',*,*,#6301,.F.);
#8510=ORIENTED_EDGE('',*,*,#6035,.F.);
#8511=ORIENTED_EDGE('',*,*,#6037,.T.);
#8512=ORIENTED_EDGE('',*,*,#6303,.T.);
#8513=ORIENTED_EDGE('',*,*,#6305,.T.);
#8514=ORIENTED_EDGE('',*,*,#6298,.T.);
#8515=ORIENTED_EDGE('',*,*,#6305,.F.);
#8516=ORIENTED_EDGE('',*,*,#6302,.F.);
#8517=ORIENTED_EDGE('',*,*,#6304,.T.);
#8518=ORIENTED_EDGE('',*,*,#6299,.T.);
#8519=ORIENTED_EDGE('',*,*,#6038,.T.);
#8520=ORIENTED_EDGE('',*,*,#6306,.F.);
#8521=ORIENTED_EDGE('',*,*,#6307,.F.);
#8522=ORIENTED_EDGE('',*,*,#6308,.T.);
#8523=ORIENTED_EDGE('',*,*,#6040,.T.);
#8524=ORIENTED_EDGE('',*,*,#6309,.T.);
#8525=ORIENTED_EDGE('',*,*,#6310,.T.);
#8526=ORIENTED_EDGE('',*,*,#6311,.F.);
#8527=ORIENTED_EDGE('',*,*,#6308,.F.);
#8528=ORIENTED_EDGE('',*,*,#6312,.F.);
#8529=ORIENTED_EDGE('',*,*,#6309,.F.);
#8530=ORIENTED_EDGE('',*,*,#6039,.F.);
#8531=ORIENTED_EDGE('',*,*,#6041,.T.);
#8532=ORIENTED_EDGE('',*,*,#6311,.T.);
#8533=ORIENTED_EDGE('',*,*,#6313,.T.);
#8534=ORIENTED_EDGE('',*,*,#6306,.T.);
#8535=ORIENTED_EDGE('',*,*,#6313,.F.);
#8536=ORIENTED_EDGE('',*,*,#6310,.F.);
#8537=ORIENTED_EDGE('',*,*,#6312,.T.);
#8538=ORIENTED_EDGE('',*,*,#6307,.T.);
#8539=ORIENTED_EDGE('',*,*,#6042,.T.);
#8540=ORIENTED_EDGE('',*,*,#6314,.F.);
#8541=ORIENTED_EDGE('',*,*,#6315,.F.);
#8542=ORIENTED_EDGE('',*,*,#6316,.T.);
#8543=ORIENTED_EDGE('',*,*,#6044,.T.);
#8544=ORIENTED_EDGE('',*,*,#6317,.T.);
#8545=ORIENTED_EDGE('',*,*,#6318,.T.);
#8546=ORIENTED_EDGE('',*,*,#6319,.F.);
#8547=ORIENTED_EDGE('',*,*,#6316,.F.);
#8548=ORIENTED_EDGE('',*,*,#6320,.F.);
#8549=ORIENTED_EDGE('',*,*,#6317,.F.);
#8550=ORIENTED_EDGE('',*,*,#6043,.F.);
#8551=ORIENTED_EDGE('',*,*,#6045,.T.);
#8552=ORIENTED_EDGE('',*,*,#6319,.T.);
#8553=ORIENTED_EDGE('',*,*,#6321,.T.);
#8554=ORIENTED_EDGE('',*,*,#6314,.T.);
#8555=ORIENTED_EDGE('',*,*,#6321,.F.);
#8556=ORIENTED_EDGE('',*,*,#6318,.F.);
#8557=ORIENTED_EDGE('',*,*,#6320,.T.);
#8558=ORIENTED_EDGE('',*,*,#6315,.T.);
#8559=ORIENTED_EDGE('',*,*,#6062,.T.);
#8560=ORIENTED_EDGE('',*,*,#6322,.F.);
#8561=ORIENTED_EDGE('',*,*,#6323,.F.);
#8562=ORIENTED_EDGE('',*,*,#6324,.T.);
#8563=ORIENTED_EDGE('',*,*,#6064,.T.);
#8564=ORIENTED_EDGE('',*,*,#6325,.T.);
#8565=ORIENTED_EDGE('',*,*,#6326,.T.);
#8566=ORIENTED_EDGE('',*,*,#6327,.F.);
#8567=ORIENTED_EDGE('',*,*,#6324,.F.);
#8568=ORIENTED_EDGE('',*,*,#6328,.F.);
#8569=ORIENTED_EDGE('',*,*,#6325,.F.);
#8570=ORIENTED_EDGE('',*,*,#6063,.F.);
#8571=ORIENTED_EDGE('',*,*,#6065,.T.);
#8572=ORIENTED_EDGE('',*,*,#6327,.T.);
#8573=ORIENTED_EDGE('',*,*,#6329,.T.);
#8574=ORIENTED_EDGE('',*,*,#6322,.T.);
#8575=ORIENTED_EDGE('',*,*,#6329,.F.);
#8576=ORIENTED_EDGE('',*,*,#6326,.F.);
#8577=ORIENTED_EDGE('',*,*,#6328,.T.);
#8578=ORIENTED_EDGE('',*,*,#6323,.T.);
#8579=ORIENTED_EDGE('',*,*,#6066,.T.);
#8580=ORIENTED_EDGE('',*,*,#6330,.F.);
#8581=ORIENTED_EDGE('',*,*,#6331,.F.);
#8582=ORIENTED_EDGE('',*,*,#6332,.T.);
#8583=ORIENTED_EDGE('',*,*,#6068,.T.);
#8584=ORIENTED_EDGE('',*,*,#6333,.T.);
#8585=ORIENTED_EDGE('',*,*,#6334,.T.);
#8586=ORIENTED_EDGE('',*,*,#6335,.F.);
#8587=ORIENTED_EDGE('',*,*,#6332,.F.);
#8588=ORIENTED_EDGE('',*,*,#6336,.F.);
#8589=ORIENTED_EDGE('',*,*,#6333,.F.);
#8590=ORIENTED_EDGE('',*,*,#6067,.F.);
#8591=ORIENTED_EDGE('',*,*,#6069,.T.);
#8592=ORIENTED_EDGE('',*,*,#6335,.T.);
#8593=ORIENTED_EDGE('',*,*,#6337,.T.);
#8594=ORIENTED_EDGE('',*,*,#6330,.T.);
#8595=ORIENTED_EDGE('',*,*,#6337,.F.);
#8596=ORIENTED_EDGE('',*,*,#6334,.F.);
#8597=ORIENTED_EDGE('',*,*,#6336,.T.);
#8598=ORIENTED_EDGE('',*,*,#6331,.T.);
#8599=ORIENTED_EDGE('',*,*,#6070,.T.);
#8600=ORIENTED_EDGE('',*,*,#6338,.F.);
#8601=ORIENTED_EDGE('',*,*,#6339,.F.);
#8602=ORIENTED_EDGE('',*,*,#6340,.T.);
#8603=ORIENTED_EDGE('',*,*,#6072,.T.);
#8604=ORIENTED_EDGE('',*,*,#6341,.T.);
#8605=ORIENTED_EDGE('',*,*,#6342,.T.);
#8606=ORIENTED_EDGE('',*,*,#6343,.F.);
#8607=ORIENTED_EDGE('',*,*,#6340,.F.);
#8608=ORIENTED_EDGE('',*,*,#6344,.F.);
#8609=ORIENTED_EDGE('',*,*,#6341,.F.);
#8610=ORIENTED_EDGE('',*,*,#6071,.F.);
#8611=ORIENTED_EDGE('',*,*,#6073,.T.);
#8612=ORIENTED_EDGE('',*,*,#6343,.T.);
#8613=ORIENTED_EDGE('',*,*,#6345,.T.);
#8614=ORIENTED_EDGE('',*,*,#6338,.T.);
#8615=ORIENTED_EDGE('',*,*,#6345,.F.);
#8616=ORIENTED_EDGE('',*,*,#6342,.F.);
#8617=ORIENTED_EDGE('',*,*,#6344,.T.);
#8618=ORIENTED_EDGE('',*,*,#6339,.T.);
#8619=ORIENTED_EDGE('',*,*,#6074,.T.);
#8620=ORIENTED_EDGE('',*,*,#6346,.F.);
#8621=ORIENTED_EDGE('',*,*,#6347,.F.);
#8622=ORIENTED_EDGE('',*,*,#6348,.T.);
#8623=ORIENTED_EDGE('',*,*,#6076,.T.);
#8624=ORIENTED_EDGE('',*,*,#6349,.T.);
#8625=ORIENTED_EDGE('',*,*,#6350,.T.);
#8626=ORIENTED_EDGE('',*,*,#6351,.F.);
#8627=ORIENTED_EDGE('',*,*,#6348,.F.);
#8628=ORIENTED_EDGE('',*,*,#6352,.F.);
#8629=ORIENTED_EDGE('',*,*,#6349,.F.);
#8630=ORIENTED_EDGE('',*,*,#6075,.F.);
#8631=ORIENTED_EDGE('',*,*,#6077,.T.);
#8632=ORIENTED_EDGE('',*,*,#6351,.T.);
#8633=ORIENTED_EDGE('',*,*,#6353,.T.);
#8634=ORIENTED_EDGE('',*,*,#6346,.T.);
#8635=ORIENTED_EDGE('',*,*,#6353,.F.);
#8636=ORIENTED_EDGE('',*,*,#6350,.F.);
#8637=ORIENTED_EDGE('',*,*,#6352,.T.);
#8638=ORIENTED_EDGE('',*,*,#6347,.T.);
#8639=ORIENTED_EDGE('',*,*,#6078,.T.);
#8640=ORIENTED_EDGE('',*,*,#6354,.F.);
#8641=ORIENTED_EDGE('',*,*,#6355,.F.);
#8642=ORIENTED_EDGE('',*,*,#6356,.T.);
#8643=ORIENTED_EDGE('',*,*,#6080,.T.);
#8644=ORIENTED_EDGE('',*,*,#6357,.T.);
#8645=ORIENTED_EDGE('',*,*,#6358,.T.);
#8646=ORIENTED_EDGE('',*,*,#6359,.F.);
#8647=ORIENTED_EDGE('',*,*,#6356,.F.);
#8648=ORIENTED_EDGE('',*,*,#6360,.F.);
#8649=ORIENTED_EDGE('',*,*,#6357,.F.);
#8650=ORIENTED_EDGE('',*,*,#6079,.F.);
#8651=ORIENTED_EDGE('',*,*,#6081,.T.);
#8652=ORIENTED_EDGE('',*,*,#6359,.T.);
#8653=ORIENTED_EDGE('',*,*,#6361,.T.);
#8654=ORIENTED_EDGE('',*,*,#6354,.T.);
#8655=ORIENTED_EDGE('',*,*,#6361,.F.);
#8656=ORIENTED_EDGE('',*,*,#6358,.F.);
#8657=ORIENTED_EDGE('',*,*,#6360,.T.);
#8658=ORIENTED_EDGE('',*,*,#6355,.T.);
#8659=ORIENTED_EDGE('',*,*,#6082,.T.);
#8660=ORIENTED_EDGE('',*,*,#6362,.F.);
#8661=ORIENTED_EDGE('',*,*,#6363,.F.);
#8662=ORIENTED_EDGE('',*,*,#6364,.T.);
#8663=ORIENTED_EDGE('',*,*,#6084,.T.);
#8664=ORIENTED_EDGE('',*,*,#6365,.T.);
#8665=ORIENTED_EDGE('',*,*,#6366,.T.);
#8666=ORIENTED_EDGE('',*,*,#6367,.F.);
#8667=ORIENTED_EDGE('',*,*,#6364,.F.);
#8668=ORIENTED_EDGE('',*,*,#6368,.F.);
#8669=ORIENTED_EDGE('',*,*,#6365,.F.);
#8670=ORIENTED_EDGE('',*,*,#6083,.F.);
#8671=ORIENTED_EDGE('',*,*,#6085,.T.);
#8672=ORIENTED_EDGE('',*,*,#6367,.T.);
#8673=ORIENTED_EDGE('',*,*,#6369,.T.);
#8674=ORIENTED_EDGE('',*,*,#6362,.T.);
#8675=ORIENTED_EDGE('',*,*,#6369,.F.);
#8676=ORIENTED_EDGE('',*,*,#6366,.F.);
#8677=ORIENTED_EDGE('',*,*,#6368,.T.);
#8678=ORIENTED_EDGE('',*,*,#6363,.T.);
#8679=ORIENTED_EDGE('',*,*,#6086,.T.);
#8680=ORIENTED_EDGE('',*,*,#6370,.F.);
#8681=ORIENTED_EDGE('',*,*,#6371,.F.);
#8682=ORIENTED_EDGE('',*,*,#6372,.T.);
#8683=ORIENTED_EDGE('',*,*,#6088,.T.);
#8684=ORIENTED_EDGE('',*,*,#6373,.T.);
#8685=ORIENTED_EDGE('',*,*,#6374,.T.);
#8686=ORIENTED_EDGE('',*,*,#6375,.F.);
#8687=ORIENTED_EDGE('',*,*,#6372,.F.);
#8688=ORIENTED_EDGE('',*,*,#6376,.F.);
#8689=ORIENTED_EDGE('',*,*,#6373,.F.);
#8690=ORIENTED_EDGE('',*,*,#6087,.F.);
#8691=ORIENTED_EDGE('',*,*,#6089,.T.);
#8692=ORIENTED_EDGE('',*,*,#6375,.T.);
#8693=ORIENTED_EDGE('',*,*,#6377,.T.);
#8694=ORIENTED_EDGE('',*,*,#6370,.T.);
#8695=ORIENTED_EDGE('',*,*,#6377,.F.);
#8696=ORIENTED_EDGE('',*,*,#6374,.F.);
#8697=ORIENTED_EDGE('',*,*,#6376,.T.);
#8698=ORIENTED_EDGE('',*,*,#6371,.T.);
#8699=ORIENTED_EDGE('',*,*,#6090,.T.);
#8700=ORIENTED_EDGE('',*,*,#6378,.F.);
#8701=ORIENTED_EDGE('',*,*,#6379,.F.);
#8702=ORIENTED_EDGE('',*,*,#6380,.T.);
#8703=ORIENTED_EDGE('',*,*,#6092,.T.);
#8704=ORIENTED_EDGE('',*,*,#6381,.T.);
#8705=ORIENTED_EDGE('',*,*,#6382,.T.);
#8706=ORIENTED_EDGE('',*,*,#6383,.F.);
#8707=ORIENTED_EDGE('',*,*,#6380,.F.);
#8708=ORIENTED_EDGE('',*,*,#6384,.F.);
#8709=ORIENTED_EDGE('',*,*,#6381,.F.);
#8710=ORIENTED_EDGE('',*,*,#6091,.F.);
#8711=ORIENTED_EDGE('',*,*,#6093,.T.);
#8712=ORIENTED_EDGE('',*,*,#6383,.T.);
#8713=ORIENTED_EDGE('',*,*,#6385,.T.);
#8714=ORIENTED_EDGE('',*,*,#6378,.T.);
#8715=ORIENTED_EDGE('',*,*,#6385,.F.);
#8716=ORIENTED_EDGE('',*,*,#6382,.F.);
#8717=ORIENTED_EDGE('',*,*,#6384,.T.);
#8718=ORIENTED_EDGE('',*,*,#6379,.T.);
#8719=ORIENTED_EDGE('',*,*,#6094,.T.);
#8720=ORIENTED_EDGE('',*,*,#6386,.F.);
#8721=ORIENTED_EDGE('',*,*,#6387,.F.);
#8722=ORIENTED_EDGE('',*,*,#6388,.T.);
#8723=ORIENTED_EDGE('',*,*,#6096,.T.);
#8724=ORIENTED_EDGE('',*,*,#6389,.T.);
#8725=ORIENTED_EDGE('',*,*,#6390,.T.);
#8726=ORIENTED_EDGE('',*,*,#6391,.F.);
#8727=ORIENTED_EDGE('',*,*,#6388,.F.);
#8728=ORIENTED_EDGE('',*,*,#6392,.F.);
#8729=ORIENTED_EDGE('',*,*,#6389,.F.);
#8730=ORIENTED_EDGE('',*,*,#6095,.F.);
#8731=ORIENTED_EDGE('',*,*,#6097,.T.);
#8732=ORIENTED_EDGE('',*,*,#6391,.T.);
#8733=ORIENTED_EDGE('',*,*,#6393,.T.);
#8734=ORIENTED_EDGE('',*,*,#6386,.T.);
#8735=ORIENTED_EDGE('',*,*,#6393,.F.);
#8736=ORIENTED_EDGE('',*,*,#6390,.F.);
#8737=ORIENTED_EDGE('',*,*,#6392,.T.);
#8738=ORIENTED_EDGE('',*,*,#6387,.T.);
#8739=ORIENTED_EDGE('',*,*,#6098,.T.);
#8740=ORIENTED_EDGE('',*,*,#6394,.F.);
#8741=ORIENTED_EDGE('',*,*,#6395,.F.);
#8742=ORIENTED_EDGE('',*,*,#6396,.T.);
#8743=ORIENTED_EDGE('',*,*,#6100,.T.);
#8744=ORIENTED_EDGE('',*,*,#6397,.T.);
#8745=ORIENTED_EDGE('',*,*,#6398,.T.);
#8746=ORIENTED_EDGE('',*,*,#6399,.F.);
#8747=ORIENTED_EDGE('',*,*,#6396,.F.);
#8748=ORIENTED_EDGE('',*,*,#6400,.F.);
#8749=ORIENTED_EDGE('',*,*,#6397,.F.);
#8750=ORIENTED_EDGE('',*,*,#6099,.F.);
#8751=ORIENTED_EDGE('',*,*,#6101,.T.);
#8752=ORIENTED_EDGE('',*,*,#6399,.T.);
#8753=ORIENTED_EDGE('',*,*,#6401,.T.);
#8754=ORIENTED_EDGE('',*,*,#6394,.T.);
#8755=ORIENTED_EDGE('',*,*,#6401,.F.);
#8756=ORIENTED_EDGE('',*,*,#6398,.F.);
#8757=ORIENTED_EDGE('',*,*,#6400,.T.);
#8758=ORIENTED_EDGE('',*,*,#6395,.T.);
#8759=ORIENTED_EDGE('',*,*,#6102,.T.);
#8760=ORIENTED_EDGE('',*,*,#6402,.F.);
#8761=ORIENTED_EDGE('',*,*,#6403,.F.);
#8762=ORIENTED_EDGE('',*,*,#6404,.T.);
#8763=ORIENTED_EDGE('',*,*,#6104,.T.);
#8764=ORIENTED_EDGE('',*,*,#6405,.T.);
#8765=ORIENTED_EDGE('',*,*,#6406,.T.);
#8766=ORIENTED_EDGE('',*,*,#6407,.F.);
#8767=ORIENTED_EDGE('',*,*,#6404,.F.);
#8768=ORIENTED_EDGE('',*,*,#6408,.F.);
#8769=ORIENTED_EDGE('',*,*,#6405,.F.);
#8770=ORIENTED_EDGE('',*,*,#6103,.F.);
#8771=ORIENTED_EDGE('',*,*,#6105,.T.);
#8772=ORIENTED_EDGE('',*,*,#6407,.T.);
#8773=ORIENTED_EDGE('',*,*,#6409,.T.);
#8774=ORIENTED_EDGE('',*,*,#6402,.T.);
#8775=ORIENTED_EDGE('',*,*,#6409,.F.);
#8776=ORIENTED_EDGE('',*,*,#6406,.F.);
#8777=ORIENTED_EDGE('',*,*,#6408,.T.);
#8778=ORIENTED_EDGE('',*,*,#6403,.T.);
#8779=ORIENTED_EDGE('',*,*,#6106,.T.);
#8780=ORIENTED_EDGE('',*,*,#6410,.F.);
#8781=ORIENTED_EDGE('',*,*,#6411,.F.);
#8782=ORIENTED_EDGE('',*,*,#6412,.T.);
#8783=ORIENTED_EDGE('',*,*,#6108,.T.);
#8784=ORIENTED_EDGE('',*,*,#6413,.T.);
#8785=ORIENTED_EDGE('',*,*,#6414,.T.);
#8786=ORIENTED_EDGE('',*,*,#6415,.F.);
#8787=ORIENTED_EDGE('',*,*,#6412,.F.);
#8788=ORIENTED_EDGE('',*,*,#6416,.F.);
#8789=ORIENTED_EDGE('',*,*,#6413,.F.);
#8790=ORIENTED_EDGE('',*,*,#6107,.F.);
#8791=ORIENTED_EDGE('',*,*,#6109,.T.);
#8792=ORIENTED_EDGE('',*,*,#6415,.T.);
#8793=ORIENTED_EDGE('',*,*,#6417,.T.);
#8794=ORIENTED_EDGE('',*,*,#6410,.T.);
#8795=ORIENTED_EDGE('',*,*,#6417,.F.);
#8796=ORIENTED_EDGE('',*,*,#6414,.F.);
#8797=ORIENTED_EDGE('',*,*,#6416,.T.);
#8798=ORIENTED_EDGE('',*,*,#6411,.T.);
#8799=ORIENTED_EDGE('',*,*,#6110,.T.);
#8800=ORIENTED_EDGE('',*,*,#6418,.F.);
#8801=ORIENTED_EDGE('',*,*,#6419,.F.);
#8802=ORIENTED_EDGE('',*,*,#6420,.T.);
#8803=ORIENTED_EDGE('',*,*,#6112,.T.);
#8804=ORIENTED_EDGE('',*,*,#6421,.T.);
#8805=ORIENTED_EDGE('',*,*,#6422,.T.);
#8806=ORIENTED_EDGE('',*,*,#6423,.F.);
#8807=ORIENTED_EDGE('',*,*,#6420,.F.);
#8808=ORIENTED_EDGE('',*,*,#6424,.F.);
#8809=ORIENTED_EDGE('',*,*,#6421,.F.);
#8810=ORIENTED_EDGE('',*,*,#6111,.F.);
#8811=ORIENTED_EDGE('',*,*,#6113,.T.);
#8812=ORIENTED_EDGE('',*,*,#6423,.T.);
#8813=ORIENTED_EDGE('',*,*,#6425,.T.);
#8814=ORIENTED_EDGE('',*,*,#6418,.T.);
#8815=ORIENTED_EDGE('',*,*,#6425,.F.);
#8816=ORIENTED_EDGE('',*,*,#6422,.F.);
#8817=ORIENTED_EDGE('',*,*,#6424,.T.);
#8818=ORIENTED_EDGE('',*,*,#6419,.T.);
#8819=ORIENTED_EDGE('',*,*,#6114,.T.);
#8820=ORIENTED_EDGE('',*,*,#6426,.F.);
#8821=ORIENTED_EDGE('',*,*,#6427,.F.);
#8822=ORIENTED_EDGE('',*,*,#6428,.T.);
#8823=ORIENTED_EDGE('',*,*,#6116,.T.);
#8824=ORIENTED_EDGE('',*,*,#6429,.T.);
#8825=ORIENTED_EDGE('',*,*,#6430,.T.);
#8826=ORIENTED_EDGE('',*,*,#6431,.F.);
#8827=ORIENTED_EDGE('',*,*,#6428,.F.);
#8828=ORIENTED_EDGE('',*,*,#6432,.F.);
#8829=ORIENTED_EDGE('',*,*,#6429,.F.);
#8830=ORIENTED_EDGE('',*,*,#6115,.F.);
#8831=ORIENTED_EDGE('',*,*,#6117,.T.);
#8832=ORIENTED_EDGE('',*,*,#6431,.T.);
#8833=ORIENTED_EDGE('',*,*,#6433,.T.);
#8834=ORIENTED_EDGE('',*,*,#6426,.T.);
#8835=ORIENTED_EDGE('',*,*,#6433,.F.);
#8836=ORIENTED_EDGE('',*,*,#6430,.F.);
#8837=ORIENTED_EDGE('',*,*,#6432,.T.);
#8838=ORIENTED_EDGE('',*,*,#6427,.T.);
#8839=ORIENTED_EDGE('',*,*,#6118,.T.);
#8840=ORIENTED_EDGE('',*,*,#6434,.F.);
#8841=ORIENTED_EDGE('',*,*,#6435,.F.);
#8842=ORIENTED_EDGE('',*,*,#6436,.T.);
#8843=ORIENTED_EDGE('',*,*,#6120,.T.);
#8844=ORIENTED_EDGE('',*,*,#6437,.T.);
#8845=ORIENTED_EDGE('',*,*,#6438,.T.);
#8846=ORIENTED_EDGE('',*,*,#6439,.F.);
#8847=ORIENTED_EDGE('',*,*,#6436,.F.);
#8848=ORIENTED_EDGE('',*,*,#6440,.F.);
#8849=ORIENTED_EDGE('',*,*,#6437,.F.);
#8850=ORIENTED_EDGE('',*,*,#6119,.F.);
#8851=ORIENTED_EDGE('',*,*,#6121,.T.);
#8852=ORIENTED_EDGE('',*,*,#6439,.T.);
#8853=ORIENTED_EDGE('',*,*,#6441,.T.);
#8854=ORIENTED_EDGE('',*,*,#6434,.T.);
#8855=ORIENTED_EDGE('',*,*,#6441,.F.);
#8856=ORIENTED_EDGE('',*,*,#6438,.F.);
#8857=ORIENTED_EDGE('',*,*,#6440,.T.);
#8858=ORIENTED_EDGE('',*,*,#6435,.T.);
#9222=CYLINDRICAL_SURFACE('',#10488,6.2);
#9223=CYLINDRICAL_SURFACE('',#10491,14.);
#9511=ADVANCED_FACE('',(#1186),#9222,.F.);
#9512=ADVANCED_FACE('',(#1187,#374,#375,#376,#377,#378,#379,#380,#381,#382,
#383,#384,#385,#386,#387,#388,#389,#390,#391,#392,#393,#394,#395,#396,#397,
#398,#399,#400,#401,#402,#403,#404,#405,#406,#407,#408,#409,#410,#411,#412),
#9223,.T.);
#9513=ADVANCED_FACE('',(#1188,#413),#651,.T.);
#9514=ADVANCED_FACE('',(#1189,#414),#652,.F.);
#9515=ADVANCED_FACE('',(#1190),#653,.T.);
#9516=ADVANCED_FACE('',(#1191),#654,.T.);
#9517=ADVANCED_FACE('',(#1192),#655,.F.);
#9518=ADVANCED_FACE('',(#1193),#656,.T.);
#9519=ADVANCED_FACE('',(#1194),#657,.T.);
#9520=ADVANCED_FACE('',(#1195),#658,.T.);
#9521=ADVANCED_FACE('',(#1196),#659,.T.);
#9522=ADVANCED_FACE('',(#1197),#660,.F.);
#9523=ADVANCED_FACE('',(#1198),#661,.T.);
#9524=ADVANCED_FACE('',(#1199),#662,.T.);
#9525=ADVANCED_FACE('',(#1200),#663,.T.);
#9526=ADVANCED_FACE('',(#1201),#664,.T.);
#9527=ADVANCED_FACE('',(#1202),#665,.F.);
#9528=ADVANCED_FACE('',(#1203),#666,.T.);
#9529=ADVANCED_FACE('',(#1204),#667,.T.);
#9530=ADVANCED_FACE('',(#1205),#668,.T.);
#9531=ADVANCED_FACE('',(#1206),#669,.T.);
#9532=ADVANCED_FACE('',(#1207),#670,.F.);
#9533=ADVANCED_FACE('',(#1208),#671,.T.);
#9534=ADVANCED_FACE('',(#1209),#672,.T.);
#9535=ADVANCED_FACE('',(#1210),#673,.T.);
#9536=ADVANCED_FACE('',(#1211),#674,.T.);
#9537=ADVANCED_FACE('',(#1212),#675,.F.);
#9538=ADVANCED_FACE('',(#1213),#676,.T.);
#9539=ADVANCED_FACE('',(#1214),#677,.T.);
#9540=ADVANCED_FACE('',(#1215),#678,.T.);
#9541=ADVANCED_FACE('',(#1216),#679,.T.);
#9542=ADVANCED_FACE('',(#1217),#680,.F.);
#9543=ADVANCED_FACE('',(#1218),#681,.T.);
#9544=ADVANCED_FACE('',(#1219),#682,.T.);
#9545=ADVANCED_FACE('',(#1220),#683,.T.);
#9546=ADVANCED_FACE('',(#1221),#684,.T.);
#9547=ADVANCED_FACE('',(#1222),#685,.F.);
#9548=ADVANCED_FACE('',(#1223),#686,.T.);
#9549=ADVANCED_FACE('',(#1224),#687,.T.);
#9550=ADVANCED_FACE('',(#1225),#688,.T.);
#9551=ADVANCED_FACE('',(#1226),#689,.T.);
#9552=ADVANCED_FACE('',(#1227),#690,.F.);
#9553=ADVANCED_FACE('',(#1228),#691,.T.);
#9554=ADVANCED_FACE('',(#1229),#692,.T.);
#9555=ADVANCED_FACE('',(#1230),#693,.T.);
#9556=ADVANCED_FACE('',(#1231),#694,.T.);
#9557=ADVANCED_FACE('',(#1232),#695,.F.);
#9558=ADVANCED_FACE('',(#1233),#696,.T.);
#9559=ADVANCED_FACE('',(#1234),#697,.T.);
#9560=ADVANCED_FACE('',(#1235),#698,.T.);
#9561=ADVANCED_FACE('',(#1236),#699,.T.);
#9562=ADVANCED_FACE('',(#1237),#700,.F.);
#9563=ADVANCED_FACE('',(#1238),#701,.T.);
#9564=ADVANCED_FACE('',(#1239),#702,.T.);
#9565=ADVANCED_FACE('',(#1240),#703,.T.);
#9566=ADVANCED_FACE('',(#1241),#704,.T.);
#9567=ADVANCED_FACE('',(#1242),#705,.F.);
#9568=ADVANCED_FACE('',(#1243),#706,.T.);
#9569=ADVANCED_FACE('',(#1244),#707,.T.);
#9570=ADVANCED_FACE('',(#1245),#708,.T.);
#9571=ADVANCED_FACE('',(#1246),#709,.T.);
#9572=ADVANCED_FACE('',(#1247),#710,.F.);
#9573=ADVANCED_FACE('',(#1248),#711,.T.);
#9574=ADVANCED_FACE('',(#1249),#712,.T.);
#9575=ADVANCED_FACE('',(#1250),#713,.T.);
#9576=ADVANCED_FACE('',(#1251),#714,.T.);
#9577=ADVANCED_FACE('',(#1252),#715,.F.);
#9578=ADVANCED_FACE('',(#1253),#716,.T.);
#9579=ADVANCED_FACE('',(#1254),#717,.T.);
#9580=ADVANCED_FACE('',(#1255),#718,.T.);
#9581=ADVANCED_FACE('',(#1256),#719,.T.);
#9582=ADVANCED_FACE('',(#1257),#720,.F.);
#9583=ADVANCED_FACE('',(#1258),#721,.T.);
#9584=ADVANCED_FACE('',(#1259),#722,.T.);
#9585=ADVANCED_FACE('',(#1260),#723,.T.);
#9586=ADVANCED_FACE('',(#1261),#724,.T.);
#9587=ADVANCED_FACE('',(#1262),#725,.F.);
#9588=ADVANCED_FACE('',(#1263),#726,.T.);
#9589=ADVANCED_FACE('',(#1264),#727,.T.);
#9590=ADVANCED_FACE('',(#1265),#728,.T.);
#9591=ADVANCED_FACE('',(#1266),#729,.T.);
#9592=ADVANCED_FACE('',(#1267),#730,.F.);
#9593=ADVANCED_FACE('',(#1268),#731,.T.);
#9594=ADVANCED_FACE('',(#1269),#732,.T.);
#9595=ADVANCED_FACE('',(#1270),#733,.T.);
#9596=ADVANCED_FACE('',(#1271),#734,.T.);
#9597=ADVANCED_FACE('',(#1272),#735,.F.);
#9598=ADVANCED_FACE('',(#1273),#736,.T.);
#9599=ADVANCED_FACE('',(#1274),#737,.T.);
#9600=ADVANCED_FACE('',(#1275),#738,.T.);
#9601=ADVANCED_FACE('',(#1276),#739,.T.);
#9602=ADVANCED_FACE('',(#1277),#740,.F.);
#9603=ADVANCED_FACE('',(#1278),#741,.T.);
#9604=ADVANCED_FACE('',(#1279),#742,.T.);
#9605=ADVANCED_FACE('',(#1280),#743,.T.);
#9606=ADVANCED_FACE('',(#1281),#744,.T.);
#9607=ADVANCED_FACE('',(#1282),#745,.F.);
#9608=ADVANCED_FACE('',(#1283),#746,.T.);
#9609=ADVANCED_FACE('',(#1284),#747,.T.);
#9610=ADVANCED_FACE('',(#1285),#748,.T.);
#9611=ADVANCED_FACE('',(#1286),#749,.T.);
#9612=ADVANCED_FACE('',(#1287),#750,.F.);
#9613=ADVANCED_FACE('',(#1288),#751,.T.);
#9614=ADVANCED_FACE('',(#1289),#752,.T.);
#9615=ADVANCED_FACE('',(#1290),#753,.T.);
#9616=ADVANCED_FACE('',(#1291),#754,.T.);
#9617=ADVANCED_FACE('',(#1292),#755,.F.);
#9618=ADVANCED_FACE('',(#1293),#756,.T.);
#9619=ADVANCED_FACE('',(#1294),#757,.T.);
#9620=ADVANCED_FACE('',(#1295),#758,.T.);
#9621=ADVANCED_FACE('',(#1296),#759,.T.);
#9622=ADVANCED_FACE('',(#1297),#760,.F.);
#9623=ADVANCED_FACE('',(#1298),#761,.T.);
#9624=ADVANCED_FACE('',(#1299),#762,.T.);
#9625=ADVANCED_FACE('',(#1300),#763,.T.);
#9626=ADVANCED_FACE('',(#1301),#764,.T.);
#9627=ADVANCED_FACE('',(#1302),#765,.F.);
#9628=ADVANCED_FACE('',(#1303),#766,.T.);
#9629=ADVANCED_FACE('',(#1304),#767,.T.);
#9630=ADVANCED_FACE('',(#1305),#768,.T.);
#9631=ADVANCED_FACE('',(#1306),#769,.T.);
#9632=ADVANCED_FACE('',(#1307),#770,.F.);
#9633=ADVANCED_FACE('',(#1308),#771,.T.);
#9634=ADVANCED_FACE('',(#1309),#772,.T.);
#9635=ADVANCED_FACE('',(#1310),#773,.T.);
#9636=ADVANCED_FACE('',(#1311),#774,.T.);
#9637=ADVANCED_FACE('',(#1312),#775,.F.);
#9638=ADVANCED_FACE('',(#1313),#776,.T.);
#9639=ADVANCED_FACE('',(#1314),#777,.T.);
#9640=ADVANCED_FACE('',(#1315),#778,.T.);
#9641=ADVANCED_FACE('',(#1316),#779,.T.);
#9642=ADVANCED_FACE('',(#1317),#780,.F.);
#9643=ADVANCED_FACE('',(#1318),#781,.T.);
#9644=ADVANCED_FACE('',(#1319),#782,.T.);
#9645=ADVANCED_FACE('',(#1320),#783,.T.);
#9646=ADVANCED_FACE('',(#1321),#784,.T.);
#9647=ADVANCED_FACE('',(#1322),#785,.F.);
#9648=ADVANCED_FACE('',(#1323),#786,.T.);
#9649=ADVANCED_FACE('',(#1324),#787,.T.);
#9650=ADVANCED_FACE('',(#1325),#788,.T.);
#9651=ADVANCED_FACE('',(#1326),#789,.T.);
#9652=ADVANCED_FACE('',(#1327),#790,.F.);
#9653=ADVANCED_FACE('',(#1328),#791,.T.);
#9654=ADVANCED_FACE('',(#1329),#792,.T.);
#9655=ADVANCED_FACE('',(#1330),#793,.T.);
#9656=ADVANCED_FACE('',(#1331),#794,.T.);
#9657=ADVANCED_FACE('',(#1332),#795,.F.);
#9658=ADVANCED_FACE('',(#1333),#796,.T.);
#9659=ADVANCED_FACE('',(#1334),#797,.T.);
#9660=ADVANCED_FACE('',(#1335),#798,.T.);
#9661=ADVANCED_FACE('',(#1336),#799,.T.);
#9662=ADVANCED_FACE('',(#1337),#800,.F.);
#9663=ADVANCED_FACE('',(#1338),#801,.T.);
#9664=ADVANCED_FACE('',(#1339),#802,.T.);
#9665=ADVANCED_FACE('',(#1340),#803,.T.);
#9666=ADVANCED_FACE('',(#1341),#804,.T.);
#9667=ADVANCED_FACE('',(#1342),#805,.F.);
#9668=ADVANCED_FACE('',(#1343),#806,.T.);
#9669=ADVANCED_FACE('',(#1344),#807,.T.);
#9670=ADVANCED_FACE('',(#1345),#808,.T.);
#9671=ADVANCED_FACE('',(#1346),#809,.T.);
#9672=ADVANCED_FACE('',(#1347),#810,.F.);
#9673=ADVANCED_FACE('',(#1348),#811,.T.);
#9674=ADVANCED_FACE('',(#1349),#812,.T.);
#9675=ADVANCED_FACE('',(#1350),#813,.T.);
#9676=ADVANCED_FACE('',(#1351),#814,.T.);
#9677=ADVANCED_FACE('',(#1352),#815,.F.);
#9678=ADVANCED_FACE('',(#1353),#816,.T.);
#9679=ADVANCED_FACE('',(#1354),#817,.T.);
#9680=ADVANCED_FACE('',(#1355),#818,.T.);
#9681=ADVANCED_FACE('',(#1356),#819,.T.);
#9682=ADVANCED_FACE('',(#1357),#820,.F.);
#9683=ADVANCED_FACE('',(#1358),#821,.T.);
#9684=ADVANCED_FACE('',(#1359),#822,.T.);
#9685=ADVANCED_FACE('',(#1360),#823,.T.);
#9686=ADVANCED_FACE('',(#1361),#824,.T.);
#9687=ADVANCED_FACE('',(#1362),#825,.F.);
#9688=ADVANCED_FACE('',(#1363),#826,.T.);
#9689=ADVANCED_FACE('',(#1364),#827,.T.);
#9690=ADVANCED_FACE('',(#1365),#828,.T.);
#9691=ADVANCED_FACE('',(#1366),#829,.T.);
#9692=ADVANCED_FACE('',(#1367),#830,.F.);
#9693=ADVANCED_FACE('',(#1368),#831,.T.);
#9694=ADVANCED_FACE('',(#1369),#832,.T.);
#9695=ADVANCED_FACE('',(#1370),#833,.T.);
#9696=ADVANCED_FACE('',(#1371),#834,.T.);
#9697=ADVANCED_FACE('',(#1372),#835,.F.);
#9698=ADVANCED_FACE('',(#1373),#836,.T.);
#9699=ADVANCED_FACE('',(#1374),#837,.T.);
#9700=ADVANCED_FACE('',(#1375),#838,.T.);
#9701=ADVANCED_FACE('',(#1376),#839,.T.);
#9702=ADVANCED_FACE('',(#1377),#840,.F.);
#9703=ADVANCED_FACE('',(#1378),#841,.T.);
#9704=ADVANCED_FACE('',(#1379),#842,.T.);
#9705=ADVANCED_FACE('',(#1380),#843,.T.);
#9706=ADVANCED_FACE('',(#1381),#844,.T.);
#9707=ADVANCED_FACE('',(#1382),#845,.F.);
#9708=ADVANCED_FACE('',(#1383),#846,.T.);
#9709=ADVANCED_FACE('',(#1384),#847,.T.);
#9710=ADVANCED_FACE('',(#1385),#848,.T.);
#9711=ADVANCED_FACE('',(#1386),#849,.T.);
#9712=ADVANCED_FACE('',(#1387),#850,.F.);
#9713=ADVANCED_FACE('',(#1388),#851,.T.);
#9714=ADVANCED_FACE('',(#1389),#852,.T.);
#9803=CLOSED_SHELL('',(#9511,#9512,#9513,#9514,#9515,#9516,#9517,#9518,
#9519,#9520,#9521,#9522,#9523,#9524,#9525,#9526,#9527,#9528,#9529,#9530,
#9531,#9532,#9533,#9534,#9535,#9536,#9537,#9538,#9539,#9540,#9541,#9542,
#9543,#9544,#9545,#9546,#9547,#9548,#9549,#9550,#9551,#9552,#9553,#9554,
#9555,#9556,#9557,#9558,#9559,#9560,#9561,#9562,#9563,#9564,#9565,#9566,
#9567,#9568,#9569,#9570,#9571,#9572,#9573,#9574,#9575,#9576,#9577,#9578,
#9579,#9580,#9581,#9582,#9583,#9584,#9585,#9586,#9587,#9588,#9589,#9590,
#9591,#9592,#9593,#9594,#9595,#9596,#9597,#9598,#9599,#9600,#9601,#9602,
#9603,#9604,#9605,#9606,#9607,#9608,#9609,#9610,#9611,#9612,#9613,#9614,
#9615,#9616,#9617,#9618,#9619,#9620,#9621,#9622,#9623,#9624,#9625,#9626,
#9627,#9628,#9629,#9630,#9631,#9632,#9633,#9634,#9635,#9636,#9637,#9638,
#9639,#9640,#9641,#9642,#9643,#9644,#9645,#9646,#9647,#9648,#9649,#9650,
#9651,#9652,#9653,#9654,#9655,#9656,#9657,#9658,#9659,#9660,#9661,#9662,
#9663,#9664,#9665,#9666,#9667,#9668,#9669,#9670,#9671,#9672,#9673,#9674,
#9675,#9676,#9677,#9678,#9679,#9680,#9681,#9682,#9683,#9684,#9685,#9686,
#9687,#9688,#9689,#9690,#9691,#9692,#9693,#9694,#9695,#9696,#9697,#9698,
#9699,#9700,#9701,#9702,#9703,#9704,#9705,#9706,#9707,#9708,#9709,#9710,
#9711,#9712,#9713,#9714));
#10487=AXIS2_PLACEMENT_3D('',#15146,#12267,#12268);
#10488=AXIS2_PLACEMENT_3D('',#15147,#12269,#12270);
#10489=AXIS2_PLACEMENT_3D('',#15149,#12271,#12272);
#10490=AXIS2_PLACEMENT_3D('',#15152,#12274,#12275);
#10491=AXIS2_PLACEMENT_3D('',#15153,#12276,#12277);
#10492=AXIS2_PLACEMENT_3D('',#15155,#12278,#12279);
#10493=AXIS2_PLACEMENT_3D('',#15159,#12281,#12282);
#10494=AXIS2_PLACEMENT_3D('',#15163,#12284,#12285);
#10495=AXIS2_PLACEMENT_3D('',#15166,#12287,#12288);
#10496=AXIS2_PLACEMENT_3D('',#15168,#12289,#12290);
#10497=AXIS2_PLACEMENT_3D('',#15171,#12292,#12293);
#10498=AXIS2_PLACEMENT_3D('',#15174,#12294,#12295);
#10499=AXIS2_PLACEMENT_3D('',#15178,#12297,#12298);
#10500=AXIS2_PLACEMENT_3D('',#15184,#12301,#12302);
#10501=AXIS2_PLACEMENT_3D('',#15187,#12304,#12305);
#10502=AXIS2_PLACEMENT_3D('',#15192,#12307,#12308);
#10503=AXIS2_PLACEMENT_3D('',#15195,#12310,#12311);
#10504=AXIS2_PLACEMENT_3D('',#15200,#12313,#12314);
#10505=AXIS2_PLACEMENT_3D('',#15203,#12316,#12317);
#10506=AXIS2_PLACEMENT_3D('',#15208,#12319,#12320);
#10507=AXIS2_PLACEMENT_3D('',#15211,#12322,#12323);
#10508=AXIS2_PLACEMENT_3D('',#15216,#12325,#12326);
#10509=AXIS2_PLACEMENT_3D('',#15219,#12328,#12329);
#10510=AXIS2_PLACEMENT_3D('',#15224,#12331,#12332);
#10511=AXIS2_PLACEMENT_3D('',#15227,#12334,#12335);
#10512=AXIS2_PLACEMENT_3D('',#15232,#12337,#12338);
#10513=AXIS2_PLACEMENT_3D('',#15235,#12340,#12341);
#10514=AXIS2_PLACEMENT_3D('',#15240,#12343,#12344);
#10515=AXIS2_PLACEMENT_3D('',#15243,#12346,#12347);
#10516=AXIS2_PLACEMENT_3D('',#15248,#12349,#12350);
#10517=AXIS2_PLACEMENT_3D('',#15251,#12352,#12353);
#10518=AXIS2_PLACEMENT_3D('',#15256,#12355,#12356);
#10519=AXIS2_PLACEMENT_3D('',#15259,#12358,#12359);
#10520=AXIS2_PLACEMENT_3D('',#15264,#12361,#12362);
#10521=AXIS2_PLACEMENT_3D('',#15267,#12364,#12365);
#10522=AXIS2_PLACEMENT_3D('',#15272,#12367,#12368);
#10523=AXIS2_PLACEMENT_3D('',#15275,#12370,#12371);
#10524=AXIS2_PLACEMENT_3D('',#15280,#12373,#12374);
#10525=AXIS2_PLACEMENT_3D('',#15283,#12376,#12377);
#10526=AXIS2_PLACEMENT_3D('',#15288,#12379,#12380);
#10527=AXIS2_PLACEMENT_3D('',#15291,#12382,#12383);
#10528=AXIS2_PLACEMENT_3D('',#15296,#12385,#12386);
#10529=AXIS2_PLACEMENT_3D('',#15299,#12388,#12389);
#10530=AXIS2_PLACEMENT_3D('',#15304,#12391,#12392);
#10531=AXIS2_PLACEMENT_3D('',#15307,#12394,#12395);
#10532=AXIS2_PLACEMENT_3D('',#15312,#12397,#12398);
#10533=AXIS2_PLACEMENT_3D('',#15315,#12400,#12401);
#10534=AXIS2_PLACEMENT_3D('',#15320,#12403,#12404);
#10535=AXIS2_PLACEMENT_3D('',#15323,#12406,#12407);
#10536=AXIS2_PLACEMENT_3D('',#15328,#12409,#12410);
#10537=AXIS2_PLACEMENT_3D('',#15331,#12412,#12413);
#10538=AXIS2_PLACEMENT_3D('',#15336,#12415,#12416);
#10539=AXIS2_PLACEMENT_3D('',#15339,#12418,#12419);
#10540=AXIS2_PLACEMENT_3D('',#15344,#12421,#12422);
#10541=AXIS2_PLACEMENT_3D('',#15347,#12424,#12425);
#10542=AXIS2_PLACEMENT_3D('',#15352,#12427,#12428);
#10543=AXIS2_PLACEMENT_3D('',#15355,#12430,#12431);
#10544=AXIS2_PLACEMENT_3D('',#15360,#12433,#12434);
#10545=AXIS2_PLACEMENT_3D('',#15363,#12436,#12437);
#10546=AXIS2_PLACEMENT_3D('',#15368,#12439,#12440);
#10547=AXIS2_PLACEMENT_3D('',#15371,#12442,#12443);
#10548=AXIS2_PLACEMENT_3D('',#15376,#12445,#12446);
#10549=AXIS2_PLACEMENT_3D('',#15379,#12448,#12449);
#10550=AXIS2_PLACEMENT_3D('',#15384,#12451,#12452);
#10551=AXIS2_PLACEMENT_3D('',#15387,#12454,#12455);
#10552=AXIS2_PLACEMENT_3D('',#15392,#12457,#12458);
#10553=AXIS2_PLACEMENT_3D('',#15395,#12460,#12461);
#10554=AXIS2_PLACEMENT_3D('',#15400,#12463,#12464);
#10555=AXIS2_PLACEMENT_3D('',#15403,#12466,#12467);
#10556=AXIS2_PLACEMENT_3D('',#15408,#12469,#12470);
#10557=AXIS2_PLACEMENT_3D('',#15411,#12472,#12473);
#10558=AXIS2_PLACEMENT_3D('',#15416,#12475,#12476);
#10559=AXIS2_PLACEMENT_3D('',#15419,#12478,#12479);
#10560=AXIS2_PLACEMENT_3D('',#15424,#12481,#12482);
#10561=AXIS2_PLACEMENT_3D('',#15427,#12484,#12485);
#10562=AXIS2_PLACEMENT_3D('',#15432,#12487,#12488);
#10563=AXIS2_PLACEMENT_3D('',#15435,#12490,#12491);
#10564=AXIS2_PLACEMENT_3D('',#15440,#12493,#12494);
#10565=AXIS2_PLACEMENT_3D('',#15443,#12496,#12497);
#10566=AXIS2_PLACEMENT_3D('',#15448,#12499,#12500);
#10567=AXIS2_PLACEMENT_3D('',#15451,#12502,#12503);
#10568=AXIS2_PLACEMENT_3D('',#15456,#12505,#12506);
#10569=AXIS2_PLACEMENT_3D('',#15459,#12508,#12509);
#10570=AXIS2_PLACEMENT_3D('',#15464,#12511,#12512);
#10571=AXIS2_PLACEMENT_3D('',#15467,#12514,#12515);
#10572=AXIS2_PLACEMENT_3D('',#15472,#12517,#12518);
#10573=AXIS2_PLACEMENT_3D('',#15475,#12520,#12521);
#10574=AXIS2_PLACEMENT_3D('',#15480,#12523,#12524);
#10575=AXIS2_PLACEMENT_3D('',#15483,#12526,#12527);
#10576=AXIS2_PLACEMENT_3D('',#15484,#12528,#12529);
#10577=AXIS2_PLACEMENT_3D('',#15485,#12530,#12531);
#10578=AXIS2_PLACEMENT_3D('',#15486,#12532,#12533);
#10579=AXIS2_PLACEMENT_3D('',#15492,#12537,#12538);
#10580=AXIS2_PLACEMENT_3D('',#15498,#12542,#12543);
#10581=AXIS2_PLACEMENT_3D('',#15500,#12545,#12546);
#10582=AXIS2_PLACEMENT_3D('',#15502,#12548,#12549);
#10583=AXIS2_PLACEMENT_3D('',#15503,#12550,#12551);
#10584=AXIS2_PLACEMENT_3D('',#15509,#12555,#12556);
#10585=AXIS2_PLACEMENT_3D('',#15515,#12560,#12561);
#10586=AXIS2_PLACEMENT_3D('',#15517,#12563,#12564);
#10587=AXIS2_PLACEMENT_3D('',#15519,#12566,#12567);
#10588=AXIS2_PLACEMENT_3D('',#15520,#12568,#12569);
#10589=AXIS2_PLACEMENT_3D('',#15526,#12573,#12574);
#10590=AXIS2_PLACEMENT_3D('',#15532,#12578,#12579);
#10591=AXIS2_PLACEMENT_3D('',#15534,#12581,#12582);
#10592=AXIS2_PLACEMENT_3D('',#15536,#12584,#12585);
#10593=AXIS2_PLACEMENT_3D('',#15537,#12586,#12587);
#10594=AXIS2_PLACEMENT_3D('',#15543,#12591,#12592);
#10595=AXIS2_PLACEMENT_3D('',#15549,#12596,#12597);
#10596=AXIS2_PLACEMENT_3D('',#15551,#12599,#12600);
#10597=AXIS2_PLACEMENT_3D('',#15553,#12602,#12603);
#10598=AXIS2_PLACEMENT_3D('',#15554,#12604,#12605);
#10599=AXIS2_PLACEMENT_3D('',#15560,#12609,#12610);
#10600=AXIS2_PLACEMENT_3D('',#15566,#12614,#12615);
#10601=AXIS2_PLACEMENT_3D('',#15568,#12617,#12618);
#10602=AXIS2_PLACEMENT_3D('',#15570,#12620,#12621);
#10603=AXIS2_PLACEMENT_3D('',#15571,#12622,#12623);
#10604=AXIS2_PLACEMENT_3D('',#15577,#12627,#12628);
#10605=AXIS2_PLACEMENT_3D('',#15583,#12632,#12633);
#10606=AXIS2_PLACEMENT_3D('',#15585,#12635,#12636);
#10607=AXIS2_PLACEMENT_3D('',#15587,#12638,#12639);
#10608=AXIS2_PLACEMENT_3D('',#15588,#12640,#12641);
#10609=AXIS2_PLACEMENT_3D('',#15594,#12645,#12646);
#10610=AXIS2_PLACEMENT_3D('',#15600,#12650,#12651);
#10611=AXIS2_PLACEMENT_3D('',#15602,#12653,#12654);
#10612=AXIS2_PLACEMENT_3D('',#15604,#12656,#12657);
#10613=AXIS2_PLACEMENT_3D('',#15605,#12658,#12659);
#10614=AXIS2_PLACEMENT_3D('',#15611,#12663,#12664);
#10615=AXIS2_PLACEMENT_3D('',#15617,#12668,#12669);
#10616=AXIS2_PLACEMENT_3D('',#15619,#12671,#12672);
#10617=AXIS2_PLACEMENT_3D('',#15621,#12674,#12675);
#10618=AXIS2_PLACEMENT_3D('',#15622,#12676,#12677);
#10619=AXIS2_PLACEMENT_3D('',#15628,#12681,#12682);
#10620=AXIS2_PLACEMENT_3D('',#15634,#12686,#12687);
#10621=AXIS2_PLACEMENT_3D('',#15636,#12689,#12690);
#10622=AXIS2_PLACEMENT_3D('',#15638,#12692,#12693);
#10623=AXIS2_PLACEMENT_3D('',#15639,#12694,#12695);
#10624=AXIS2_PLACEMENT_3D('',#15645,#12699,#12700);
#10625=AXIS2_PLACEMENT_3D('',#15651,#12704,#12705);
#10626=AXIS2_PLACEMENT_3D('',#15653,#12707,#12708);
#10627=AXIS2_PLACEMENT_3D('',#15655,#12710,#12711);
#10628=AXIS2_PLACEMENT_3D('',#15656,#12712,#12713);
#10629=AXIS2_PLACEMENT_3D('',#15662,#12717,#12718);
#10630=AXIS2_PLACEMENT_3D('',#15668,#12722,#12723);
#10631=AXIS2_PLACEMENT_3D('',#15670,#12725,#12726);
#10632=AXIS2_PLACEMENT_3D('',#15672,#12728,#12729);
#10633=AXIS2_PLACEMENT_3D('',#15673,#12730,#12731);
#10634=AXIS2_PLACEMENT_3D('',#15679,#12735,#12736);
#10635=AXIS2_PLACEMENT_3D('',#15685,#12740,#12741);
#10636=AXIS2_PLACEMENT_3D('',#15687,#12743,#12744);
#10637=AXIS2_PLACEMENT_3D('',#15689,#12746,#12747);
#10638=AXIS2_PLACEMENT_3D('',#15690,#12748,#12749);
#10639=AXIS2_PLACEMENT_3D('',#15696,#12753,#12754);
#10640=AXIS2_PLACEMENT_3D('',#15702,#12758,#12759);
#10641=AXIS2_PLACEMENT_3D('',#15704,#12761,#12762);
#10642=AXIS2_PLACEMENT_3D('',#15706,#12764,#12765);
#10643=AXIS2_PLACEMENT_3D('',#15707,#12766,#12767);
#10644=AXIS2_PLACEMENT_3D('',#15713,#12771,#12772);
#10645=AXIS2_PLACEMENT_3D('',#15719,#12776,#12777);
#10646=AXIS2_PLACEMENT_3D('',#15721,#12779,#12780);
#10647=AXIS2_PLACEMENT_3D('',#15723,#12782,#12783);
#10648=AXIS2_PLACEMENT_3D('',#15724,#12784,#12785);
#10649=AXIS2_PLACEMENT_3D('',#15730,#12789,#12790);
#10650=AXIS2_PLACEMENT_3D('',#15736,#12794,#12795);
#10651=AXIS2_PLACEMENT_3D('',#15738,#12797,#12798);
#10652=AXIS2_PLACEMENT_3D('',#15740,#12800,#12801);
#10653=AXIS2_PLACEMENT_3D('',#15741,#12802,#12803);
#10654=AXIS2_PLACEMENT_3D('',#15747,#12807,#12808);
#10655=AXIS2_PLACEMENT_3D('',#15753,#12812,#12813);
#10656=AXIS2_PLACEMENT_3D('',#15755,#12815,#12816);
#10657=AXIS2_PLACEMENT_3D('',#15757,#12818,#12819);
#10658=AXIS2_PLACEMENT_3D('',#15758,#12820,#12821);
#10659=AXIS2_PLACEMENT_3D('',#15764,#12825,#12826);
#10660=AXIS2_PLACEMENT_3D('',#15770,#12830,#12831);
#10661=AXIS2_PLACEMENT_3D('',#15772,#12833,#12834);
#10662=AXIS2_PLACEMENT_3D('',#15774,#12836,#12837);
#10663=AXIS2_PLACEMENT_3D('',#15775,#12838,#12839);
#10664=AXIS2_PLACEMENT_3D('',#15781,#12843,#12844);
#10665=AXIS2_PLACEMENT_3D('',#15787,#12848,#12849);
#10666=AXIS2_PLACEMENT_3D('',#15789,#12851,#12852);
#10667=AXIS2_PLACEMENT_3D('',#15791,#12854,#12855);
#10668=AXIS2_PLACEMENT_3D('',#15792,#12856,#12857);
#10669=AXIS2_PLACEMENT_3D('',#15798,#12861,#12862);
#10670=AXIS2_PLACEMENT_3D('',#15804,#12866,#12867);
#10671=AXIS2_PLACEMENT_3D('',#15806,#12869,#12870);
#10672=AXIS2_PLACEMENT_3D('',#15808,#12872,#12873);
#10673=AXIS2_PLACEMENT_3D('',#15809,#12874,#12875);
#10674=AXIS2_PLACEMENT_3D('',#15815,#12879,#12880);
#10675=AXIS2_PLACEMENT_3D('',#15821,#12884,#12885);
#10676=AXIS2_PLACEMENT_3D('',#15823,#12887,#12888);
#10677=AXIS2_PLACEMENT_3D('',#15825,#12890,#12891);
#10678=AXIS2_PLACEMENT_3D('',#15826,#12892,#12893);
#10679=AXIS2_PLACEMENT_3D('',#15832,#12897,#12898);
#10680=AXIS2_PLACEMENT_3D('',#15838,#12902,#12903);
#10681=AXIS2_PLACEMENT_3D('',#15840,#12905,#12906);
#10682=AXIS2_PLACEMENT_3D('',#15842,#12908,#12909);
#10683=AXIS2_PLACEMENT_3D('',#15843,#12910,#12911);
#10684=AXIS2_PLACEMENT_3D('',#15849,#12915,#12916);
#10685=AXIS2_PLACEMENT_3D('',#15855,#12920,#12921);
#10686=AXIS2_PLACEMENT_3D('',#15857,#12923,#12924);
#10687=AXIS2_PLACEMENT_3D('',#15859,#12926,#12927);
#10688=AXIS2_PLACEMENT_3D('',#15860,#12928,#12929);
#10689=AXIS2_PLACEMENT_3D('',#15866,#12933,#12934);
#10690=AXIS2_PLACEMENT_3D('',#15872,#12938,#12939);
#10691=AXIS2_PLACEMENT_3D('',#15874,#12941,#12942);
#10692=AXIS2_PLACEMENT_3D('',#15876,#12944,#12945);
#10693=AXIS2_PLACEMENT_3D('',#15877,#12946,#12947);
#10694=AXIS2_PLACEMENT_3D('',#15883,#12951,#12952);
#10695=AXIS2_PLACEMENT_3D('',#15889,#12956,#12957);
#10696=AXIS2_PLACEMENT_3D('',#15891,#12959,#12960);
#10697=AXIS2_PLACEMENT_3D('',#15893,#12962,#12963);
#10698=AXIS2_PLACEMENT_3D('',#15894,#12964,#12965);
#10699=AXIS2_PLACEMENT_3D('',#15900,#12969,#12970);
#10700=AXIS2_PLACEMENT_3D('',#15906,#12974,#12975);
#10701=AXIS2_PLACEMENT_3D('',#15908,#12977,#12978);
#10702=AXIS2_PLACEMENT_3D('',#15910,#12980,#12981);
#10703=AXIS2_PLACEMENT_3D('',#15911,#12982,#12983);
#10704=AXIS2_PLACEMENT_3D('',#15917,#12987,#12988);
#10705=AXIS2_PLACEMENT_3D('',#15923,#12992,#12993);
#10706=AXIS2_PLACEMENT_3D('',#15925,#12995,#12996);
#10707=AXIS2_PLACEMENT_3D('',#15927,#12998,#12999);
#10708=AXIS2_PLACEMENT_3D('',#15928,#13000,#13001);
#10709=AXIS2_PLACEMENT_3D('',#15934,#13005,#13006);
#10710=AXIS2_PLACEMENT_3D('',#15940,#13010,#13011);
#10711=AXIS2_PLACEMENT_3D('',#15942,#13013,#13014);
#10712=AXIS2_PLACEMENT_3D('',#15944,#13016,#13017);
#10713=AXIS2_PLACEMENT_3D('',#15945,#13018,#13019);
#10714=AXIS2_PLACEMENT_3D('',#15951,#13023,#13024);
#10715=AXIS2_PLACEMENT_3D('',#15957,#13028,#13029);
#10716=AXIS2_PLACEMENT_3D('',#15959,#13031,#13032);
#10717=AXIS2_PLACEMENT_3D('',#15961,#13034,#13035);
#10718=AXIS2_PLACEMENT_3D('',#15962,#13036,#13037);
#10719=AXIS2_PLACEMENT_3D('',#15968,#13041,#13042);
#10720=AXIS2_PLACEMENT_3D('',#15974,#13046,#13047);
#10721=AXIS2_PLACEMENT_3D('',#15976,#13049,#13050);
#10722=AXIS2_PLACEMENT_3D('',#15978,#13052,#13053);
#10723=AXIS2_PLACEMENT_3D('',#15979,#13054,#13055);
#10724=AXIS2_PLACEMENT_3D('',#15985,#13059,#13060);
#10725=AXIS2_PLACEMENT_3D('',#15991,#13064,#13065);
#10726=AXIS2_PLACEMENT_3D('',#15993,#13067,#13068);
#10727=AXIS2_PLACEMENT_3D('',#15995,#13070,#13071);
#10728=AXIS2_PLACEMENT_3D('',#15996,#13072,#13073);
#10729=AXIS2_PLACEMENT_3D('',#16002,#13077,#13078);
#10730=AXIS2_PLACEMENT_3D('',#16008,#13082,#13083);
#10731=AXIS2_PLACEMENT_3D('',#16010,#13085,#13086);
#10732=AXIS2_PLACEMENT_3D('',#16012,#13088,#13089);
#10733=AXIS2_PLACEMENT_3D('',#16013,#13090,#13091);
#10734=AXIS2_PLACEMENT_3D('',#16019,#13095,#13096);
#10735=AXIS2_PLACEMENT_3D('',#16025,#13100,#13101);
#10736=AXIS2_PLACEMENT_3D('',#16027,#13103,#13104);
#10737=AXIS2_PLACEMENT_3D('',#16029,#13106,#13107);
#10738=AXIS2_PLACEMENT_3D('',#16030,#13108,#13109);
#10739=AXIS2_PLACEMENT_3D('',#16036,#13113,#13114);
#10740=AXIS2_PLACEMENT_3D('',#16042,#13118,#13119);
#10741=AXIS2_PLACEMENT_3D('',#16044,#13121,#13122);
#10742=AXIS2_PLACEMENT_3D('',#16046,#13124,#13125);
#10743=AXIS2_PLACEMENT_3D('',#16047,#13126,#13127);
#10744=AXIS2_PLACEMENT_3D('',#16053,#13131,#13132);
#10745=AXIS2_PLACEMENT_3D('',#16059,#13136,#13137);
#10746=AXIS2_PLACEMENT_3D('',#16061,#13139,#13140);
#10747=AXIS2_PLACEMENT_3D('',#16063,#13142,#13143);
#10748=AXIS2_PLACEMENT_3D('',#16064,#13144,#13145);
#10749=AXIS2_PLACEMENT_3D('',#16070,#13149,#13150);
#10750=AXIS2_PLACEMENT_3D('',#16076,#13154,#13155);
#10751=AXIS2_PLACEMENT_3D('',#16078,#13157,#13158);
#10752=AXIS2_PLACEMENT_3D('',#16080,#13160,#13161);
#10753=AXIS2_PLACEMENT_3D('',#16081,#13162,#13163);
#10754=AXIS2_PLACEMENT_3D('',#16087,#13167,#13168);
#10755=AXIS2_PLACEMENT_3D('',#16093,#13172,#13173);
#10756=AXIS2_PLACEMENT_3D('',#16095,#13175,#13176);
#10757=AXIS2_PLACEMENT_3D('',#16097,#13178,#13179);
#10758=AXIS2_PLACEMENT_3D('',#16098,#13180,#13181);
#10759=AXIS2_PLACEMENT_3D('',#16104,#13185,#13186);
#10760=AXIS2_PLACEMENT_3D('',#16110,#13190,#13191);
#10761=AXIS2_PLACEMENT_3D('',#16112,#13193,#13194);
#10762=AXIS2_PLACEMENT_3D('',#16114,#13196,#13197);
#10763=AXIS2_PLACEMENT_3D('',#16115,#13198,#13199);
#10764=AXIS2_PLACEMENT_3D('',#16121,#13203,#13204);
#10765=AXIS2_PLACEMENT_3D('',#16127,#13208,#13209);
#10766=AXIS2_PLACEMENT_3D('',#16129,#13211,#13212);
#10767=AXIS2_PLACEMENT_3D('',#16131,#13214,#13215);
#10768=AXIS2_PLACEMENT_3D('',#16132,#13216,#13217);
#10769=AXIS2_PLACEMENT_3D('',#16138,#13221,#13222);
#10770=AXIS2_PLACEMENT_3D('',#16144,#13226,#13227);
#10771=AXIS2_PLACEMENT_3D('',#16146,#13229,#13230);
#10772=AXIS2_PLACEMENT_3D('',#16148,#13232,#13233);
#10773=AXIS2_PLACEMENT_3D('',#16149,#13234,#13235);
#10774=AXIS2_PLACEMENT_3D('',#16155,#13239,#13240);
#10775=AXIS2_PLACEMENT_3D('',#16161,#13244,#13245);
#10776=AXIS2_PLACEMENT_3D('',#16163,#13247,#13248);
#10777=AXIS2_PLACEMENT_3D('',#16165,#13250,#13251);
#12267=DIRECTION('axis',(0.,0.,1.));
#12268=DIRECTION('refdir',(1.,0.,0.));
#12269=DIRECTION('center_axis',(0.,0.,-1.));
#12270=DIRECTION('ref_axis',(-1.,0.,0.));
#12271=DIRECTION('center_axis',(0.,0.,1.));
#12272=DIRECTION('ref_axis',(1.,0.,0.));
#12273=DIRECTION('',(0.,0.,-1.));
#12274=DIRECTION('center_axis',(0.,0.,1.));
#12275=DIRECTION('ref_axis',(1.,0.,0.));
#12276=DIRECTION('center_axis',(0.,0.,-1.));
#12277=DIRECTION('ref_axis',(-1.,0.,0.));
#12278=DIRECTION('center_axis',(0.,0.,1.));
#12279=DIRECTION('ref_axis',(1.,0.,0.));
#12280=DIRECTION('',(0.,0.,1.));
#12281=DIRECTION('center_axis',(0.,0.,1.));
#12282=DIRECTION('ref_axis',(1.,0.,0.));
#12283=DIRECTION('',(0.,0.,-1.));
#12284=DIRECTION('center_axis',(0.,0.,1.));
#12285=DIRECTION('ref_axis',(1.,0.,0.));
#12286=DIRECTION('',(0.,0.,1.));
#12287=DIRECTION('center_axis',(0.,0.,1.));
#12288=DIRECTION('ref_axis',(1.,0.,0.));
#12289=DIRECTION('center_axis',(0.,0.,1.));
#12290=DIRECTION('ref_axis',(1.,0.,0.));
#12291=DIRECTION('',(0.,0.,1.));
#12292=DIRECTION('center_axis',(0.,0.,1.));
#12293=DIRECTION('ref_axis',(1.,0.,0.));
#12294=DIRECTION('center_axis',(0.,0.,1.));
#12295=DIRECTION('ref_axis',(1.,0.,0.));
#12296=DIRECTION('',(0.,0.,1.));
#12297=DIRECTION('center_axis',(0.,0.,1.));
#12298=DIRECTION('ref_axis',(1.,0.,0.));
#12299=DIRECTION('',(0.,0.,-1.));
#12300=DIRECTION('',(0.,0.,-1.));
#12301=DIRECTION('center_axis',(0.,0.,1.));
#12302=DIRECTION('ref_axis',(1.,0.,0.));
#12303=DIRECTION('',(0.,0.,1.));
#12304=DIRECTION('center_axis',(0.,0.,1.));
#12305=DIRECTION('ref_axis',(1.,0.,0.));
#12306=DIRECTION('',(0.,0.,-1.));
#12307=DIRECTION('center_axis',(0.,0.,1.));
#12308=DIRECTION('ref_axis',(1.,0.,0.));
#12309=DIRECTION('',(0.,0.,1.));
#12310=DIRECTION('center_axis',(0.,0.,1.));
#12311=DIRECTION('ref_axis',(1.,0.,0.));
#12312=DIRECTION('',(0.,0.,-1.));
#12313=DIRECTION('center_axis',(0.,0.,1.));
#12314=DIRECTION('ref_axis',(1.,0.,0.));
#12315=DIRECTION('',(0.,0.,1.));
#12316=DIRECTION('center_axis',(0.,0.,1.));
#12317=DIRECTION('ref_axis',(1.,0.,0.));
#12318=DIRECTION('',(0.,0.,-1.));
#12319=DIRECTION('center_axis',(0.,0.,1.));
#12320=DIRECTION('ref_axis',(1.,0.,0.));
#12321=DIRECTION('',(0.,0.,1.));
#12322=DIRECTION('center_axis',(0.,0.,1.));
#12323=DIRECTION('ref_axis',(1.,0.,0.));
#12324=DIRECTION('',(0.,0.,-1.));
#12325=DIRECTION('center_axis',(0.,0.,1.));
#12326=DIRECTION('ref_axis',(1.,0.,0.));
#12327=DIRECTION('',(0.,0.,1.));
#12328=DIRECTION('center_axis',(0.,0.,1.));
#12329=DIRECTION('ref_axis',(1.,0.,0.));
#12330=DIRECTION('',(0.,0.,-1.));
#12331=DIRECTION('center_axis',(0.,0.,1.));
#12332=DIRECTION('ref_axis',(1.,0.,0.));
#12333=DIRECTION('',(0.,0.,1.));
#12334=DIRECTION('center_axis',(0.,0.,1.));
#12335=DIRECTION('ref_axis',(1.,0.,0.));
#12336=DIRECTION('',(0.,0.,-1.));
#12337=DIRECTION('center_axis',(0.,0.,1.));
#12338=DIRECTION('ref_axis',(1.,0.,0.));
#12339=DIRECTION('',(0.,0.,1.));
#12340=DIRECTION('center_axis',(0.,0.,1.));
#12341=DIRECTION('ref_axis',(1.,0.,0.));
#12342=DIRECTION('',(0.,0.,-1.));
#12343=DIRECTION('center_axis',(0.,0.,1.));
#12344=DIRECTION('ref_axis',(1.,0.,0.));
#12345=DIRECTION('',(0.,0.,1.));
#12346=DIRECTION('center_axis',(0.,0.,1.));
#12347=DIRECTION('ref_axis',(1.,0.,0.));
#12348=DIRECTION('',(0.,0.,-1.));
#12349=DIRECTION('center_axis',(0.,0.,1.));
#12350=DIRECTION('ref_axis',(1.,0.,0.));
#12351=DIRECTION('',(0.,0.,1.));
#12352=DIRECTION('center_axis',(0.,0.,1.));
#12353=DIRECTION('ref_axis',(1.,0.,0.));
#12354=DIRECTION('',(0.,0.,-1.));
#12355=DIRECTION('center_axis',(0.,0.,1.));
#12356=DIRECTION('ref_axis',(1.,0.,0.));
#12357=DIRECTION('',(0.,0.,1.));
#12358=DIRECTION('center_axis',(0.,0.,1.));
#12359=DIRECTION('ref_axis',(1.,0.,0.));
#12360=DIRECTION('',(0.,0.,-1.));
#12361=DIRECTION('center_axis',(0.,0.,1.));
#12362=DIRECTION('ref_axis',(1.,0.,0.));
#12363=DIRECTION('',(0.,0.,1.));
#12364=DIRECTION('center_axis',(0.,0.,1.));
#12365=DIRECTION('ref_axis',(1.,0.,0.));
#12366=DIRECTION('',(0.,0.,-1.));
#12367=DIRECTION('center_axis',(0.,0.,1.));
#12368=DIRECTION('ref_axis',(1.,0.,0.));
#12369=DIRECTION('',(0.,0.,1.));
#12370=DIRECTION('center_axis',(0.,0.,1.));
#12371=DIRECTION('ref_axis',(1.,0.,0.));
#12372=DIRECTION('',(0.,0.,-1.));
#12373=DIRECTION('center_axis',(0.,0.,1.));
#12374=DIRECTION('ref_axis',(1.,0.,0.));
#12375=DIRECTION('',(0.,0.,1.));
#12376=DIRECTION('center_axis',(0.,0.,1.));
#12377=DIRECTION('ref_axis',(1.,0.,0.));
#12378=DIRECTION('',(0.,0.,-1.));
#12379=DIRECTION('center_axis',(0.,0.,1.));
#12380=DIRECTION('ref_axis',(1.,0.,0.));
#12381=DIRECTION('',(0.,0.,1.));
#12382=DIRECTION('center_axis',(0.,0.,1.));
#12383=DIRECTION('ref_axis',(1.,0.,0.));
#12384=DIRECTION('',(0.,0.,-1.));
#12385=DIRECTION('center_axis',(0.,0.,1.));
#12386=DIRECTION('ref_axis',(1.,0.,0.));
#12387=DIRECTION('',(0.,0.,1.));
#12388=DIRECTION('center_axis',(0.,0.,1.));
#12389=DIRECTION('ref_axis',(1.,0.,0.));
#12390=DIRECTION('',(0.,0.,-1.));
#12391=DIRECTION('center_axis',(0.,0.,1.));
#12392=DIRECTION('ref_axis',(1.,0.,0.));
#12393=DIRECTION('',(0.,0.,1.));
#12394=DIRECTION('center_axis',(0.,0.,1.));
#12395=DIRECTION('ref_axis',(1.,0.,0.));
#12396=DIRECTION('',(0.,0.,-1.));
#12397=DIRECTION('center_axis',(0.,0.,1.));
#12398=DIRECTION('ref_axis',(1.,0.,0.));
#12399=DIRECTION('',(0.,0.,1.));
#12400=DIRECTION('center_axis',(0.,0.,1.));
#12401=DIRECTION('ref_axis',(1.,0.,0.));
#12402=DIRECTION('',(0.,0.,-1.));
#12403=DIRECTION('center_axis',(0.,0.,1.));
#12404=DIRECTION('ref_axis',(1.,0.,0.));
#12405=DIRECTION('',(0.,0.,1.));
#12406=DIRECTION('center_axis',(0.,0.,1.));
#12407=DIRECTION('ref_axis',(1.,0.,0.));
#12408=DIRECTION('',(0.,0.,-1.));
#12409=DIRECTION('center_axis',(0.,0.,1.));
#12410=DIRECTION('ref_axis',(1.,0.,0.));
#12411=DIRECTION('',(0.,0.,1.));
#12412=DIRECTION('center_axis',(0.,0.,1.));
#12413=DIRECTION('ref_axis',(1.,0.,0.));
#12414=DIRECTION('',(0.,0.,-1.));
#12415=DIRECTION('center_axis',(0.,0.,1.));
#12416=DIRECTION('ref_axis',(1.,0.,0.));
#12417=DIRECTION('',(0.,0.,1.));
#12418=DIRECTION('center_axis',(0.,0.,1.));
#12419=DIRECTION('ref_axis',(1.,0.,0.));
#12420=DIRECTION('',(0.,0.,-1.));
#12421=DIRECTION('center_axis',(0.,0.,1.));
#12422=DIRECTION('ref_axis',(1.,0.,0.));
#12423=DIRECTION('',(0.,0.,1.));
#12424=DIRECTION('center_axis',(0.,0.,1.));
#12425=DIRECTION('ref_axis',(1.,0.,0.));
#12426=DIRECTION('',(0.,0.,-1.));
#12427=DIRECTION('center_axis',(0.,0.,1.));
#12428=DIRECTION('ref_axis',(1.,0.,0.));
#12429=DIRECTION('',(0.,0.,1.));
#12430=DIRECTION('center_axis',(0.,0.,1.));
#12431=DIRECTION('ref_axis',(1.,0.,0.));
#12432=DIRECTION('',(0.,0.,-1.));
#12433=DIRECTION('center_axis',(0.,0.,1.));
#12434=DIRECTION('ref_axis',(1.,0.,0.));
#12435=DIRECTION('',(0.,0.,1.));
#12436=DIRECTION('center_axis',(0.,0.,1.));
#12437=DIRECTION('ref_axis',(1.,0.,0.));
#12438=DIRECTION('',(0.,0.,-1.));
#12439=DIRECTION('center_axis',(0.,0.,1.));
#12440=DIRECTION('ref_axis',(1.,0.,0.));
#12441=DIRECTION('',(0.,0.,1.));
#12442=DIRECTION('center_axis',(0.,0.,1.));
#12443=DIRECTION('ref_axis',(1.,0.,0.));
#12444=DIRECTION('',(0.,0.,-1.));
#12445=DIRECTION('center_axis',(0.,0.,1.));
#12446=DIRECTION('ref_axis',(1.,0.,0.));
#12447=DIRECTION('',(0.,0.,1.));
#12448=DIRECTION('center_axis',(0.,0.,1.));
#12449=DIRECTION('ref_axis',(1.,0.,0.));
#12450=DIRECTION('',(0.,0.,-1.));
#12451=DIRECTION('center_axis',(0.,0.,1.));
#12452=DIRECTION('ref_axis',(1.,0.,0.));
#12453=DIRECTION('',(0.,0.,1.));
#12454=DIRECTION('center_axis',(0.,0.,1.));
#12455=DIRECTION('ref_axis',(1.,0.,0.));
#12456=DIRECTION('',(0.,0.,-1.));
#12457=DIRECTION('center_axis',(0.,0.,1.));
#12458=DIRECTION('ref_axis',(1.,0.,0.));
#12459=DIRECTION('',(0.,0.,1.));
#12460=DIRECTION('center_axis',(0.,0.,1.));
#12461=DIRECTION('ref_axis',(1.,0.,0.));
#12462=DIRECTION('',(0.,0.,-1.));
#12463=DIRECTION('center_axis',(0.,0.,1.));
#12464=DIRECTION('ref_axis',(1.,0.,0.));
#12465=DIRECTION('',(0.,0.,1.));
#12466=DIRECTION('center_axis',(0.,0.,1.));
#12467=DIRECTION('ref_axis',(1.,0.,0.));
#12468=DIRECTION('',(0.,0.,-1.));
#12469=DIRECTION('center_axis',(0.,0.,1.));
#12470=DIRECTION('ref_axis',(1.,0.,0.));
#12471=DIRECTION('',(0.,0.,1.));
#12472=DIRECTION('center_axis',(0.,0.,1.));
#12473=DIRECTION('ref_axis',(1.,0.,0.));
#12474=DIRECTION('',(0.,0.,-1.));
#12475=DIRECTION('center_axis',(0.,0.,1.));
#12476=DIRECTION('ref_axis',(1.,0.,0.));
#12477=DIRECTION('',(0.,0.,1.));
#12478=DIRECTION('center_axis',(0.,0.,1.));
#12479=DIRECTION('ref_axis',(1.,0.,0.));
#12480=DIRECTION('',(0.,0.,-1.));
#12481=DIRECTION('center_axis',(0.,0.,1.));
#12482=DIRECTION('ref_axis',(1.,0.,0.));
#12483=DIRECTION('',(0.,0.,1.));
#12484=DIRECTION('center_axis',(0.,0.,1.));
#12485=DIRECTION('ref_axis',(1.,0.,0.));
#12486=DIRECTION('',(0.,0.,-1.));
#12487=DIRECTION('center_axis',(0.,0.,1.));
#12488=DIRECTION('ref_axis',(1.,0.,0.));
#12489=DIRECTION('',(0.,0.,1.));
#12490=DIRECTION('center_axis',(0.,0.,1.));
#12491=DIRECTION('ref_axis',(1.,0.,0.));
#12492=DIRECTION('',(0.,0.,-1.));
#12493=DIRECTION('center_axis',(0.,0.,1.));
#12494=DIRECTION('ref_axis',(1.,0.,0.));
#12495=DIRECTION('',(0.,0.,1.));
#12496=DIRECTION('center_axis',(0.,0.,1.));
#12497=DIRECTION('ref_axis',(1.,0.,0.));
#12498=DIRECTION('',(0.,0.,-1.));
#12499=DIRECTION('center_axis',(0.,0.,1.));
#12500=DIRECTION('ref_axis',(1.,0.,0.));
#12501=DIRECTION('',(0.,0.,1.));
#12502=DIRECTION('center_axis',(0.,0.,1.));
#12503=DIRECTION('ref_axis',(1.,0.,0.));
#12504=DIRECTION('',(0.,0.,-1.));
#12505=DIRECTION('center_axis',(0.,0.,1.));
#12506=DIRECTION('ref_axis',(1.,0.,0.));
#12507=DIRECTION('',(0.,0.,1.));
#12508=DIRECTION('center_axis',(0.,0.,1.));
#12509=DIRECTION('ref_axis',(1.,0.,0.));
#12510=DIRECTION('',(0.,0.,-1.));
#12511=DIRECTION('center_axis',(0.,0.,1.));
#12512=DIRECTION('ref_axis',(1.,0.,0.));
#12513=DIRECTION('',(0.,0.,1.));
#12514=DIRECTION('center_axis',(0.,0.,1.));
#12515=DIRECTION('ref_axis',(1.,0.,0.));
#12516=DIRECTION('',(0.,0.,-1.));
#12517=DIRECTION('center_axis',(0.,0.,1.));
#12518=DIRECTION('ref_axis',(1.,0.,0.));
#12519=DIRECTION('',(0.,0.,1.));
#12520=DIRECTION('center_axis',(0.,0.,1.));
#12521=DIRECTION('ref_axis',(1.,0.,0.));
#12522=DIRECTION('',(0.,0.,-1.));
#12523=DIRECTION('center_axis',(0.,0.,1.));
#12524=DIRECTION('ref_axis',(1.,0.,0.));
#12525=DIRECTION('',(0.,0.,1.));
#12526=DIRECTION('center_axis',(0.,0.,1.));
#12527=DIRECTION('ref_axis',(1.,0.,0.));
#12528=DIRECTION('center_axis',(0.,0.,1.));
#12529=DIRECTION('ref_axis',(1.,0.,0.));
#12530=DIRECTION('center_axis',(0.,0.,1.));
#12531=DIRECTION('ref_axis',(1.,0.,0.));
#12532=DIRECTION('center_axis',(0.707106781186547,0.707106781186548,0.));
#12533=DIRECTION('ref_axis',(-0.707106781186548,0.707106781186547,0.));
#12534=DIRECTION('',(0.707106781186548,-0.707106781186546,0.));
#12535=DIRECTION('',(0.,0.,-1.));
#12536=DIRECTION('',(0.707106781186548,-0.707106781186546,0.));
#12537=DIRECTION('center_axis',(-0.707106781186548,-0.707106781186547,0.));
#12538=DIRECTION('ref_axis',(0.707106781186547,-0.707106781186548,0.));
#12539=DIRECTION('',(-0.707106781186547,0.707106781186549,0.));
#12540=DIRECTION('',(0.,0.,-1.));
#12541=DIRECTION('',(-0.707106781186547,0.707106781186549,0.));
#12542=DIRECTION('center_axis',(0.,0.,1.));
#12543=DIRECTION('ref_axis',(1.,0.,0.));
#12544=DIRECTION('',(-0.707106781186547,-0.707106781186547,0.));
#12545=DIRECTION('center_axis',(0.,0.,1.));
#12546=DIRECTION('ref_axis',(1.,0.,0.));
#12547=DIRECTION('',(-0.707106781186547,-0.707106781186547,0.));
#12548=DIRECTION('center_axis',(0.707106781186548,-0.707106781186548,0.));
#12549=DIRECTION('ref_axis',(0.707106781186548,0.707106781186548,0.));
#12550=DIRECTION('center_axis',(1.,-1.80700362080917E-16,0.));
#12551=DIRECTION('ref_axis',(1.80700362080917E-16,1.,0.));
#12552=DIRECTION('',(-1.80700362080917E-16,-1.,0.));
#12553=DIRECTION('',(0.,0.,-1.));
#12554=DIRECTION('',(-1.80700362080917E-16,-1.,0.));
#12555=DIRECTION('center_axis',(-1.,1.80700362080917E-16,0.));
#12556=DIRECTION('ref_axis',(-1.80700362080917E-16,-1.,0.));
#12557=DIRECTION('',(1.80700362080917E-16,1.,0.));
#12558=DIRECTION('',(0.,0.,-1.));
#12559=DIRECTION('',(1.80700362080917E-16,1.,0.));
#12560=DIRECTION('center_axis',(0.,0.,1.));
#12561=DIRECTION('ref_axis',(1.,0.,0.));
#12562=DIRECTION('',(-1.,0.,0.));
#12563=DIRECTION('center_axis',(0.,0.,1.));
#12564=DIRECTION('ref_axis',(1.,0.,0.));
#12565=DIRECTION('',(-1.,0.,0.));
#12566=DIRECTION('center_axis',(0.,-1.,0.));
#12567=DIRECTION('ref_axis',(0.,0.,-1.));
#12568=DIRECTION('center_axis',(0.707106781186548,-0.707106781186547,0.));
#12569=DIRECTION('ref_axis',(0.707106781186547,0.707106781186548,0.));
#12570=DIRECTION('',(-0.707106781186547,-0.707106781186549,0.));
#12571=DIRECTION('',(0.,0.,-1.));
#12572=DIRECTION('',(-0.707106781186547,-0.707106781186549,0.));
#12573=DIRECTION('center_axis',(-0.707106781186547,0.707106781186548,0.));
#12574=DIRECTION('ref_axis',(-0.707106781186548,-0.707106781186547,0.));
#12575=DIRECTION('',(0.707106781186548,0.707106781186546,0.));
#12576=DIRECTION('',(0.,0.,-1.));
#12577=DIRECTION('',(0.707106781186548,0.707106781186546,0.));
#12578=DIRECTION('center_axis',(0.,0.,1.));
#12579=DIRECTION('ref_axis',(1.,0.,0.));
#12580=DIRECTION('',(-0.707106781186547,0.707106781186547,0.));
#12581=DIRECTION('center_axis',(0.,0.,1.));
#12582=DIRECTION('ref_axis',(1.,0.,0.));
#12583=DIRECTION('',(-0.707106781186547,0.707106781186547,0.));
#12584=DIRECTION('center_axis',(-0.707106781186548,-0.707106781186548,0.));
#12585=DIRECTION('ref_axis',(0.707106781186548,-0.707106781186548,0.));
#12586=DIRECTION('center_axis',(-1.35525271560688E-16,-1.,0.));
#12587=DIRECTION('ref_axis',(1.,-1.35525271560688E-16,0.));
#12588=DIRECTION('',(-1.,1.35525271560688E-16,0.));
#12589=DIRECTION('',(0.,0.,-1.));
#12590=DIRECTION('',(-1.,1.35525271560688E-16,0.));
#12591=DIRECTION('center_axis',(1.20466908053945E-16,1.,0.));
#12592=DIRECTION('ref_axis',(-1.,1.20466908053945E-16,0.));
#12593=DIRECTION('',(1.,-1.20466908053945E-16,0.));
#12594=DIRECTION('',(0.,0.,-1.));
#12595=DIRECTION('',(1.,-1.20466908053945E-16,0.));
#12596=DIRECTION('center_axis',(0.,0.,1.));
#12597=DIRECTION('ref_axis',(1.,0.,0.));
#12598=DIRECTION('',(0.,1.,0.));
#12599=DIRECTION('center_axis',(0.,0.,1.));
#12600=DIRECTION('ref_axis',(1.,0.,0.));
#12601=DIRECTION('',(0.,1.,0.));
#12602=DIRECTION('center_axis',(-1.,0.,0.));
#12603=DIRECTION('ref_axis',(0.,0.,1.));
#12604=DIRECTION('center_axis',(-0.707106781186547,-0.707106781186548,0.));
#12605=DIRECTION('ref_axis',(0.707106781186548,-0.707106781186547,0.));
#12606=DIRECTION('',(-0.707106781186548,0.707106781186546,0.));
#12607=DIRECTION('',(0.,0.,-1.));
#12608=DIRECTION('',(-0.707106781186548,0.707106781186546,0.));
#12609=DIRECTION('center_axis',(0.707106781186548,0.707106781186547,0.));
#12610=DIRECTION('ref_axis',(-0.707106781186547,0.707106781186548,0.));
#12611=DIRECTION('',(0.707106781186547,-0.707106781186549,0.));
#12612=DIRECTION('',(0.,0.,-1.));
#12613=DIRECTION('',(0.707106781186547,-0.707106781186549,0.));
#12614=DIRECTION('center_axis',(0.,0.,1.));
#12615=DIRECTION('ref_axis',(1.,0.,0.));
#12616=DIRECTION('',(0.707106781186547,0.707106781186547,0.));
#12617=DIRECTION('center_axis',(0.,0.,1.));
#12618=DIRECTION('ref_axis',(1.,0.,0.));
#12619=DIRECTION('',(0.707106781186547,0.707106781186547,0.));
#12620=DIRECTION('center_axis',(-0.707106781186548,0.707106781186548,0.));
#12621=DIRECTION('ref_axis',(-0.707106781186548,-0.707106781186548,0.));
#12622=DIRECTION('center_axis',(-1.,6.02334540269724E-17,0.));
#12623=DIRECTION('ref_axis',(-6.02334540269724E-17,-1.,0.));
#12624=DIRECTION('',(6.02334540269724E-17,1.,0.));
#12625=DIRECTION('',(0.,0.,-1.));
#12626=DIRECTION('',(6.02334540269724E-17,1.,0.));
#12627=DIRECTION('center_axis',(1.,-6.02334540269724E-17,0.));
#12628=DIRECTION('ref_axis',(6.02334540269724E-17,1.,0.));
#12629=DIRECTION('',(-6.02334540269724E-17,-1.,0.));
#12630=DIRECTION('',(0.,0.,-1.));
#12631=DIRECTION('',(-6.02334540269724E-17,-1.,0.));
#12632=DIRECTION('center_axis',(0.,0.,1.));
#12633=DIRECTION('ref_axis',(1.,0.,0.));
#12634=DIRECTION('',(1.,0.,0.));
#12635=DIRECTION('center_axis',(0.,0.,1.));
#12636=DIRECTION('ref_axis',(1.,0.,0.));
#12637=DIRECTION('',(1.,0.,0.));
#12638=DIRECTION('center_axis',(0.,1.,0.));
#12639=DIRECTION('ref_axis',(0.,0.,1.));
#12640=DIRECTION('center_axis',(-0.707106781186548,0.707106781186547,0.));
#12641=DIRECTION('ref_axis',(-0.707106781186547,-0.707106781186548,0.));
#12642=DIRECTION('',(0.707106781186547,0.707106781186549,0.));
#12643=DIRECTION('',(0.,0.,-1.));
#12644=DIRECTION('',(0.707106781186547,0.707106781186549,0.));
#12645=DIRECTION('center_axis',(0.707106781186547,-0.707106781186548,0.));
#12646=DIRECTION('ref_axis',(0.707106781186548,0.707106781186547,0.));
#12647=DIRECTION('',(-0.707106781186548,-0.707106781186546,0.));
#12648=DIRECTION('',(0.,0.,-1.));
#12649=DIRECTION('',(-0.707106781186548,-0.707106781186546,0.));
#12650=DIRECTION('center_axis',(0.,0.,1.));
#12651=DIRECTION('ref_axis',(1.,0.,0.));
#12652=DIRECTION('',(0.707106781186547,-0.707106781186547,0.));
#12653=DIRECTION('center_axis',(0.,0.,1.));
#12654=DIRECTION('ref_axis',(1.,0.,0.));
#12655=DIRECTION('',(0.707106781186547,-0.707106781186547,0.));
#12656=DIRECTION('center_axis',(0.707106781186548,0.707106781186548,0.));
#12657=DIRECTION('ref_axis',(-0.707106781186548,0.707106781186548,0.));
#12658=DIRECTION('center_axis',(0.,1.,0.));
#12659=DIRECTION('ref_axis',(0.,0.,1.));
#12660=DIRECTION('',(1.,0.,0.));
#12661=DIRECTION('',(0.,0.,-1.));
#12662=DIRECTION('',(1.,0.,0.));
#12663=DIRECTION('center_axis',(0.,-1.,0.));
#12664=DIRECTION('ref_axis',(0.,0.,-1.));
#12665=DIRECTION('',(-1.,0.,0.));
#12666=DIRECTION('',(0.,0.,-1.));
#12667=DIRECTION('',(-1.,0.,0.));
#12668=DIRECTION('center_axis',(0.,0.,1.));
#12669=DIRECTION('ref_axis',(1.,0.,0.));
#12670=DIRECTION('',(0.,-1.,0.));
#12671=DIRECTION('center_axis',(0.,0.,1.));
#12672=DIRECTION('ref_axis',(1.,0.,0.));
#12673=DIRECTION('',(0.,-1.,0.));
#12674=DIRECTION('center_axis',(1.,0.,0.));
#12675=DIRECTION('ref_axis',(0.,0.,-1.));
#12676=DIRECTION('center_axis',(-0.156434465040231,0.987688340595138,0.));
#12677=DIRECTION('ref_axis',(-0.987688340595138,-0.156434465040231,0.));
#12678=DIRECTION('',(0.987688340595138,0.156434465040231,0.));
#12679=DIRECTION('',(0.,0.,-1.));
#12680=DIRECTION('',(0.987688340595138,0.156434465040231,0.));
#12681=DIRECTION('center_axis',(0.156434465040231,-0.987688340595138,0.));
#12682=DIRECTION('ref_axis',(0.987688340595138,0.156434465040231,0.));
#12683=DIRECTION('',(-0.987688340595138,-0.156434465040231,0.));
#12684=DIRECTION('',(0.,0.,-1.));
#12685=DIRECTION('',(-0.987688340595138,-0.156434465040231,0.));
#12686=DIRECTION('center_axis',(0.,0.,1.));
#12687=DIRECTION('ref_axis',(1.,0.,0.));
#12688=DIRECTION('',(0.156434465040223,-0.987688340595139,0.));
#12689=DIRECTION('center_axis',(0.,0.,1.));
#12690=DIRECTION('ref_axis',(1.,0.,0.));
#12691=DIRECTION('',(0.156434465040223,-0.987688340595139,0.));
#12692=DIRECTION('center_axis',(0.987688340595139,0.156434465040223,0.));
#12693=DIRECTION('ref_axis',(-0.156434465040223,0.987688340595139,0.));
#12694=DIRECTION('center_axis',(0.156434465040232,0.987688340595138,0.));
#12695=DIRECTION('ref_axis',(-0.987688340595138,0.156434465040232,0.));
#12696=DIRECTION('',(0.987688340595138,-0.156434465040232,0.));
#12697=DIRECTION('',(0.,0.,-1.));
#12698=DIRECTION('',(0.987688340595138,-0.156434465040232,0.));
#12699=DIRECTION('center_axis',(-0.156434465040231,-0.987688340595138,0.));
#12700=DIRECTION('ref_axis',(0.987688340595138,-0.156434465040231,0.));
#12701=DIRECTION('',(-0.987688340595138,0.156434465040231,0.));
#12702=DIRECTION('',(0.,0.,-1.));
#12703=DIRECTION('',(-0.987688340595138,0.156434465040231,0.));
#12704=DIRECTION('center_axis',(0.,0.,1.));
#12705=DIRECTION('ref_axis',(1.,0.,0.));
#12706=DIRECTION('',(-0.156434465040224,-0.987688340595139,0.));
#12707=DIRECTION('center_axis',(0.,0.,1.));
#12708=DIRECTION('ref_axis',(1.,0.,0.));
#12709=DIRECTION('',(-0.156434465040224,-0.987688340595139,0.));
#12710=DIRECTION('center_axis',(0.987688340595139,-0.156434465040224,0.));
#12711=DIRECTION('ref_axis',(0.156434465040224,0.987688340595139,0.));
#12712=DIRECTION('center_axis',(0.309016994374948,0.951056516295154,0.));
#12713=DIRECTION('ref_axis',(-0.951056516295154,0.309016994374948,0.));
#12714=DIRECTION('',(0.951056516295153,-0.309016994374948,0.));
#12715=DIRECTION('',(0.,0.,-1.));
#12716=DIRECTION('',(0.951056516295153,-0.309016994374948,0.));
#12717=DIRECTION('center_axis',(-0.309016994374947,-0.951056516295154,0.));
#12718=DIRECTION('ref_axis',(0.951056516295154,-0.309016994374947,0.));
#12719=DIRECTION('',(-0.951056516295154,0.309016994374947,0.));
#12720=DIRECTION('',(0.,0.,-1.));
#12721=DIRECTION('',(-0.951056516295154,0.309016994374947,0.));
#12722=DIRECTION('center_axis',(0.,0.,1.));
#12723=DIRECTION('ref_axis',(1.,0.,0.));
#12724=DIRECTION('',(-0.309016994374941,-0.951056516295156,0.));
#12725=DIRECTION('center_axis',(0.,0.,1.));
#12726=DIRECTION('ref_axis',(1.,0.,0.));
#12727=DIRECTION('',(-0.309016994374941,-0.951056516295156,0.));
#12728=DIRECTION('center_axis',(0.951056516295156,-0.309016994374941,0.));
#12729=DIRECTION('ref_axis',(0.309016994374941,0.951056516295156,0.));
#12730=DIRECTION('center_axis',(0.453990499739548,0.891006524188367,0.));
#12731=DIRECTION('ref_axis',(-0.891006524188367,0.453990499739548,0.));
#12732=DIRECTION('',(0.891006524188367,-0.453990499739548,0.));
#12733=DIRECTION('',(0.,0.,-1.));
#12734=DIRECTION('',(0.891006524188367,-0.453990499739548,0.));
#12735=DIRECTION('center_axis',(-0.453990499739548,-0.891006524188367,0.));
#12736=DIRECTION('ref_axis',(0.891006524188367,-0.453990499739548,0.));
#12737=DIRECTION('',(-0.891006524188367,0.453990499739548,0.));
#12738=DIRECTION('',(0.,0.,-1.));
#12739=DIRECTION('',(-0.891006524188367,0.453990499739548,0.));
#12740=DIRECTION('center_axis',(0.,0.,1.));
#12741=DIRECTION('ref_axis',(1.,0.,0.));
#12742=DIRECTION('',(-0.453990499739554,-0.891006524188364,0.));
#12743=DIRECTION('center_axis',(0.,0.,1.));
#12744=DIRECTION('ref_axis',(1.,0.,0.));
#12745=DIRECTION('',(-0.453990499739554,-0.891006524188364,0.));
#12746=DIRECTION('center_axis',(0.891006524188364,-0.453990499739554,0.));
#12747=DIRECTION('ref_axis',(0.453990499739554,0.891006524188364,0.));
#12748=DIRECTION('center_axis',(0.587785252292473,0.809016994374947,0.));
#12749=DIRECTION('ref_axis',(-0.809016994374947,0.587785252292473,0.));
#12750=DIRECTION('',(0.809016994374947,-0.587785252292473,0.));
#12751=DIRECTION('',(0.,0.,-1.));
#12752=DIRECTION('',(0.809016994374947,-0.587785252292473,0.));
#12753=DIRECTION('center_axis',(-0.587785252292474,-0.809016994374946,0.));
#12754=DIRECTION('ref_axis',(0.809016994374946,-0.587785252292474,0.));
#12755=DIRECTION('',(-0.809016994374946,0.587785252292474,0.));
#12756=DIRECTION('',(0.,0.,-1.));
#12757=DIRECTION('',(-0.809016994374946,0.587785252292474,0.));
#12758=DIRECTION('center_axis',(0.,0.,1.));
#12759=DIRECTION('ref_axis',(1.,0.,0.));
#12760=DIRECTION('',(-0.587785252292475,-0.809016994374946,0.));
#12761=DIRECTION('center_axis',(0.,0.,1.));
#12762=DIRECTION('ref_axis',(1.,0.,0.));
#12763=DIRECTION('',(-0.587785252292475,-0.809016994374946,0.));
#12764=DIRECTION('center_axis',(0.809016994374946,-0.587785252292475,0.));
#12765=DIRECTION('ref_axis',(0.587785252292475,0.809016994374946,0.));
#12766=DIRECTION('center_axis',(0.809016994374948,0.587785252292472,0.));
#12767=DIRECTION('ref_axis',(-0.587785252292472,0.809016994374948,0.));
#12768=DIRECTION('',(0.587785252292472,-0.809016994374948,0.));
#12769=DIRECTION('',(0.,0.,-1.));
#12770=DIRECTION('',(0.587785252292472,-0.809016994374948,0.));
#12771=DIRECTION('center_axis',(-0.809016994374948,-0.587785252292472,0.));
#12772=DIRECTION('ref_axis',(0.587785252292472,-0.809016994374948,0.));
#12773=DIRECTION('',(-0.587785252292472,0.809016994374948,0.));
#12774=DIRECTION('',(0.,0.,-1.));
#12775=DIRECTION('',(-0.587785252292472,0.809016994374948,0.));
#12776=DIRECTION('center_axis',(0.,0.,1.));
#12777=DIRECTION('ref_axis',(1.,0.,0.));
#12778=DIRECTION('',(-0.809016994374946,-0.587785252292475,0.));
#12779=DIRECTION('center_axis',(0.,0.,1.));
#12780=DIRECTION('ref_axis',(1.,0.,0.));
#12781=DIRECTION('',(-0.809016994374946,-0.587785252292475,0.));
#12782=DIRECTION('center_axis',(0.587785252292475,-0.809016994374946,0.));
#12783=DIRECTION('ref_axis',(0.809016994374946,0.587785252292475,0.));
#12784=DIRECTION('center_axis',(0.891006524188367,0.453990499739548,0.));
#12785=DIRECTION('ref_axis',(-0.453990499739548,0.891006524188367,0.));
#12786=DIRECTION('',(0.453990499739548,-0.891006524188367,0.));
#12787=DIRECTION('',(0.,0.,-1.));
#12788=DIRECTION('',(0.453990499739548,-0.891006524188367,0.));
#12789=DIRECTION('center_axis',(-0.891006524188367,-0.453990499739548,0.));
#12790=DIRECTION('ref_axis',(0.453990499739548,-0.891006524188367,0.));
#12791=DIRECTION('',(-0.453990499739548,0.891006524188367,0.));
#12792=DIRECTION('',(0.,0.,-1.));
#12793=DIRECTION('',(-0.453990499739548,0.891006524188367,0.));
#12794=DIRECTION('center_axis',(0.,0.,1.));
#12795=DIRECTION('ref_axis',(1.,0.,0.));
#12796=DIRECTION('',(-0.891006524188364,-0.453990499739554,0.));
#12797=DIRECTION('center_axis',(0.,0.,1.));
#12798=DIRECTION('ref_axis',(1.,0.,0.));
#12799=DIRECTION('',(-0.891006524188364,-0.453990499739554,0.));
#12800=DIRECTION('center_axis',(0.453990499739554,-0.891006524188364,0.));
#12801=DIRECTION('ref_axis',(0.891006524188364,0.453990499739554,0.));
#12802=DIRECTION('center_axis',(0.951056516295154,0.309016994374947,0.));
#12803=DIRECTION('ref_axis',(-0.309016994374947,0.951056516295154,0.));
#12804=DIRECTION('',(0.309016994374947,-0.951056516295154,0.));
#12805=DIRECTION('',(0.,0.,-1.));
#12806=DIRECTION('',(0.309016994374947,-0.951056516295154,0.));
#12807=DIRECTION('center_axis',(-0.951056516295154,-0.309016994374947,0.));
#12808=DIRECTION('ref_axis',(0.309016994374947,-0.951056516295154,0.));
#12809=DIRECTION('',(-0.309016994374947,0.951056516295154,0.));
#12810=DIRECTION('',(0.,0.,-1.));
#12811=DIRECTION('',(-0.309016994374947,0.951056516295154,0.));
#12812=DIRECTION('center_axis',(0.,0.,1.));
#12813=DIRECTION('ref_axis',(1.,0.,0.));
#12814=DIRECTION('',(-0.951056516295156,-0.309016994374941,0.));
#12815=DIRECTION('center_axis',(0.,0.,1.));
#12816=DIRECTION('ref_axis',(1.,0.,0.));
#12817=DIRECTION('',(-0.951056516295156,-0.309016994374941,0.));
#12818=DIRECTION('center_axis',(0.309016994374941,-0.951056516295156,0.));
#12819=DIRECTION('ref_axis',(0.951056516295156,0.309016994374941,0.));
#12820=DIRECTION('center_axis',(0.987688340595138,0.156434465040231,0.));
#12821=DIRECTION('ref_axis',(-0.156434465040231,0.987688340595138,0.));
#12822=DIRECTION('',(0.156434465040231,-0.987688340595138,0.));
#12823=DIRECTION('',(0.,0.,-1.));
#12824=DIRECTION('',(0.156434465040231,-0.987688340595138,0.));
#12825=DIRECTION('center_axis',(-0.987688340595138,-0.156434465040231,0.));
#12826=DIRECTION('ref_axis',(0.156434465040231,-0.987688340595138,0.));
#12827=DIRECTION('',(-0.156434465040231,0.987688340595138,0.));
#12828=DIRECTION('',(0.,0.,-1.));
#12829=DIRECTION('',(-0.156434465040231,0.987688340595138,0.));
#12830=DIRECTION('center_axis',(0.,0.,1.));
#12831=DIRECTION('ref_axis',(1.,0.,0.));
#12832=DIRECTION('',(-0.987688340595139,-0.156434465040223,0.));
#12833=DIRECTION('center_axis',(0.,0.,1.));
#12834=DIRECTION('ref_axis',(1.,0.,0.));
#12835=DIRECTION('',(-0.987688340595139,-0.156434465040223,0.));
#12836=DIRECTION('center_axis',(0.156434465040223,-0.987688340595139,0.));
#12837=DIRECTION('ref_axis',(0.987688340595139,0.156434465040223,0.));
#12838=DIRECTION('center_axis',(0.987688340595138,-0.156434465040231,0.));
#12839=DIRECTION('ref_axis',(0.156434465040231,0.987688340595138,0.));
#12840=DIRECTION('',(-0.156434465040231,-0.987688340595138,0.));
#12841=DIRECTION('',(0.,0.,-1.));
#12842=DIRECTION('',(-0.156434465040231,-0.987688340595138,0.));
#12843=DIRECTION('center_axis',(-0.987688340595138,0.156434465040231,0.));
#12844=DIRECTION('ref_axis',(-0.156434465040231,-0.987688340595138,0.));
#12845=DIRECTION('',(0.156434465040231,0.987688340595138,0.));
#12846=DIRECTION('',(0.,0.,-1.));
#12847=DIRECTION('',(0.156434465040231,0.987688340595138,0.));
#12848=DIRECTION('center_axis',(0.,0.,1.));
#12849=DIRECTION('ref_axis',(1.,0.,0.));
#12850=DIRECTION('',(-0.987688340595139,0.156434465040224,0.));
#12851=DIRECTION('center_axis',(0.,0.,1.));
#12852=DIRECTION('ref_axis',(1.,0.,0.));
#12853=DIRECTION('',(-0.987688340595139,0.156434465040224,0.));
#12854=DIRECTION('center_axis',(-0.156434465040224,-0.987688340595139,0.));
#12855=DIRECTION('ref_axis',(0.987688340595139,-0.156434465040224,0.));
#12856=DIRECTION('center_axis',(0.951056516295154,-0.309016994374948,0.));
#12857=DIRECTION('ref_axis',(0.309016994374948,0.951056516295154,0.));
#12858=DIRECTION('',(-0.309016994374948,-0.951056516295153,0.));
#12859=DIRECTION('',(0.,0.,-1.));
#12860=DIRECTION('',(-0.309016994374948,-0.951056516295153,0.));
#12861=DIRECTION('center_axis',(-0.951056516295154,0.309016994374947,0.));
#12862=DIRECTION('ref_axis',(-0.309016994374947,-0.951056516295154,0.));
#12863=DIRECTION('',(0.309016994374947,0.951056516295154,0.));
#12864=DIRECTION('',(0.,0.,-1.));
#12865=DIRECTION('',(0.309016994374947,0.951056516295154,0.));
#12866=DIRECTION('center_axis',(0.,0.,1.));
#12867=DIRECTION('ref_axis',(1.,0.,0.));
#12868=DIRECTION('',(-0.951056516295156,0.309016994374941,0.));
#12869=DIRECTION('center_axis',(0.,0.,1.));
#12870=DIRECTION('ref_axis',(1.,0.,0.));
#12871=DIRECTION('',(-0.951056516295156,0.309016994374941,0.));
#12872=DIRECTION('center_axis',(-0.309016994374941,-0.951056516295156,0.));
#12873=DIRECTION('ref_axis',(0.951056516295156,-0.309016994374941,0.));
#12874=DIRECTION('center_axis',(0.891006524188367,-0.453990499739548,0.));
#12875=DIRECTION('ref_axis',(0.453990499739548,0.891006524188367,0.));
#12876=DIRECTION('',(-0.453990499739548,-0.891006524188367,0.));
#12877=DIRECTION('',(0.,0.,-1.));
#12878=DIRECTION('',(-0.453990499739548,-0.891006524188367,0.));
#12879=DIRECTION('center_axis',(-0.891006524188367,0.453990499739548,0.));
#12880=DIRECTION('ref_axis',(-0.453990499739548,-0.891006524188367,0.));
#12881=DIRECTION('',(0.453990499739548,0.891006524188367,0.));
#12882=DIRECTION('',(0.,0.,-1.));
#12883=DIRECTION('',(0.453990499739548,0.891006524188367,0.));
#12884=DIRECTION('center_axis',(0.,0.,1.));
#12885=DIRECTION('ref_axis',(1.,0.,0.));
#12886=DIRECTION('',(-0.891006524188364,0.453990499739554,0.));
#12887=DIRECTION('center_axis',(0.,0.,1.));
#12888=DIRECTION('ref_axis',(1.,0.,0.));
#12889=DIRECTION('',(-0.891006524188364,0.453990499739554,0.));
#12890=DIRECTION('center_axis',(-0.453990499739554,-0.891006524188364,0.));
#12891=DIRECTION('ref_axis',(0.891006524188364,-0.453990499739554,0.));
#12892=DIRECTION('center_axis',(0.809016994374947,-0.587785252292473,0.));
#12893=DIRECTION('ref_axis',(0.587785252292473,0.809016994374947,0.));
#12894=DIRECTION('',(-0.587785252292473,-0.809016994374947,0.));
#12895=DIRECTION('',(0.,0.,-1.));
#12896=DIRECTION('',(-0.587785252292473,-0.809016994374947,0.));
#12897=DIRECTION('center_axis',(-0.809016994374946,0.587785252292474,0.));
#12898=DIRECTION('ref_axis',(-0.587785252292474,-0.809016994374946,0.));
#12899=DIRECTION('',(0.587785252292474,0.809016994374946,0.));
#12900=DIRECTION('',(0.,0.,-1.));
#12901=DIRECTION('',(0.587785252292474,0.809016994374946,0.));
#12902=DIRECTION('center_axis',(0.,0.,1.));
#12903=DIRECTION('ref_axis',(1.,0.,0.));
#12904=DIRECTION('',(-0.809016994374946,0.587785252292475,0.));
#12905=DIRECTION('center_axis',(0.,0.,1.));
#12906=DIRECTION('ref_axis',(1.,0.,0.));
#12907=DIRECTION('',(-0.809016994374946,0.587785252292475,0.));
#12908=DIRECTION('center_axis',(-0.587785252292475,-0.809016994374946,0.));
#12909=DIRECTION('ref_axis',(0.809016994374946,-0.587785252292475,0.));
#12910=DIRECTION('center_axis',(0.587785252292472,-0.809016994374948,0.));
#12911=DIRECTION('ref_axis',(0.809016994374948,0.587785252292472,0.));
#12912=DIRECTION('',(-0.809016994374948,-0.587785252292472,0.));
#12913=DIRECTION('',(0.,0.,-1.));
#12914=DIRECTION('',(-0.809016994374948,-0.587785252292472,0.));
#12915=DIRECTION('center_axis',(-0.587785252292472,0.809016994374948,0.));
#12916=DIRECTION('ref_axis',(-0.809016994374948,-0.587785252292472,0.));
#12917=DIRECTION('',(0.809016994374948,0.587785252292472,0.));
#12918=DIRECTION('',(0.,0.,-1.));
#12919=DIRECTION('',(0.809016994374948,0.587785252292472,0.));
#12920=DIRECTION('center_axis',(0.,0.,1.));
#12921=DIRECTION('ref_axis',(1.,0.,0.));
#12922=DIRECTION('',(-0.587785252292475,0.809016994374946,0.));
#12923=DIRECTION('center_axis',(0.,0.,1.));
#12924=DIRECTION('ref_axis',(1.,0.,0.));
#12925=DIRECTION('',(-0.587785252292475,0.809016994374946,0.));
#12926=DIRECTION('center_axis',(-0.809016994374946,-0.587785252292475,0.));
#12927=DIRECTION('ref_axis',(0.587785252292475,-0.809016994374946,0.));
#12928=DIRECTION('center_axis',(0.453990499739548,-0.891006524188367,0.));
#12929=DIRECTION('ref_axis',(0.891006524188367,0.453990499739548,0.));
#12930=DIRECTION('',(-0.891006524188367,-0.453990499739548,0.));
#12931=DIRECTION('',(0.,0.,-1.));
#12932=DIRECTION('',(-0.891006524188367,-0.453990499739548,0.));
#12933=DIRECTION('center_axis',(-0.453990499739548,0.891006524188367,0.));
#12934=DIRECTION('ref_axis',(-0.891006524188367,-0.453990499739548,0.));
#12935=DIRECTION('',(0.891006524188367,0.453990499739548,0.));
#12936=DIRECTION('',(0.,0.,-1.));
#12937=DIRECTION('',(0.891006524188367,0.453990499739548,0.));
#12938=DIRECTION('center_axis',(0.,0.,1.));
#12939=DIRECTION('ref_axis',(1.,0.,0.));
#12940=DIRECTION('',(-0.453990499739554,0.891006524188364,0.));
#12941=DIRECTION('center_axis',(0.,0.,1.));
#12942=DIRECTION('ref_axis',(1.,0.,0.));
#12943=DIRECTION('',(-0.453990499739554,0.891006524188364,0.));
#12944=DIRECTION('center_axis',(-0.891006524188364,-0.453990499739554,0.));
#12945=DIRECTION('ref_axis',(0.453990499739554,-0.891006524188364,0.));
#12946=DIRECTION('center_axis',(0.309016994374947,-0.951056516295154,0.));
#12947=DIRECTION('ref_axis',(0.951056516295154,0.309016994374947,0.));
#12948=DIRECTION('',(-0.951056516295154,-0.309016994374947,0.));
#12949=DIRECTION('',(0.,0.,-1.));
#12950=DIRECTION('',(-0.951056516295154,-0.309016994374947,0.));
#12951=DIRECTION('center_axis',(-0.309016994374947,0.951056516295154,0.));
#12952=DIRECTION('ref_axis',(-0.951056516295154,-0.309016994374947,0.));
#12953=DIRECTION('',(0.951056516295154,0.309016994374947,0.));
#12954=DIRECTION('',(0.,0.,-1.));
#12955=DIRECTION('',(0.951056516295154,0.309016994374947,0.));
#12956=DIRECTION('center_axis',(0.,0.,1.));
#12957=DIRECTION('ref_axis',(1.,0.,0.));
#12958=DIRECTION('',(-0.309016994374941,0.951056516295156,0.));
#12959=DIRECTION('center_axis',(0.,0.,1.));
#12960=DIRECTION('ref_axis',(1.,0.,0.));
#12961=DIRECTION('',(-0.309016994374941,0.951056516295156,0.));
#12962=DIRECTION('center_axis',(-0.951056516295156,-0.309016994374941,0.));
#12963=DIRECTION('ref_axis',(0.309016994374941,-0.951056516295156,0.));
#12964=DIRECTION('center_axis',(0.156434465040231,-0.987688340595138,0.));
#12965=DIRECTION('ref_axis',(0.987688340595138,0.156434465040231,0.));
#12966=DIRECTION('',(-0.987688340595138,-0.156434465040231,0.));
#12967=DIRECTION('',(0.,0.,-1.));
#12968=DIRECTION('',(-0.987688340595138,-0.156434465040231,0.));
#12969=DIRECTION('center_axis',(-0.156434465040231,0.987688340595138,0.));
#12970=DIRECTION('ref_axis',(-0.987688340595138,-0.156434465040231,0.));
#12971=DIRECTION('',(0.987688340595138,0.156434465040231,0.));
#12972=DIRECTION('',(0.,0.,-1.));
#12973=DIRECTION('',(0.987688340595138,0.156434465040231,0.));
#12974=DIRECTION('center_axis',(0.,0.,1.));
#12975=DIRECTION('ref_axis',(1.,0.,0.));
#12976=DIRECTION('',(-0.156434465040223,0.987688340595139,0.));
#12977=DIRECTION('center_axis',(0.,0.,1.));
#12978=DIRECTION('ref_axis',(1.,0.,0.));
#12979=DIRECTION('',(-0.156434465040223,0.987688340595139,0.));
#12980=DIRECTION('center_axis',(-0.987688340595139,-0.156434465040223,0.));
#12981=DIRECTION('ref_axis',(0.156434465040223,-0.987688340595139,0.));
#12982=DIRECTION('center_axis',(-0.156434465040231,-0.987688340595138,0.));
#12983=DIRECTION('ref_axis',(0.987688340595138,-0.156434465040231,0.));
#12984=DIRECTION('',(-0.987688340595138,0.156434465040231,0.));
#12985=DIRECTION('',(0.,0.,-1.));
#12986=DIRECTION('',(-0.987688340595138,0.156434465040231,0.));
#12987=DIRECTION('center_axis',(0.156434465040231,0.987688340595138,0.));
#12988=DIRECTION('ref_axis',(-0.987688340595138,0.156434465040231,0.));
#12989=DIRECTION('',(0.987688340595138,-0.156434465040231,0.));
#12990=DIRECTION('',(0.,0.,-1.));
#12991=DIRECTION('',(0.987688340595138,-0.156434465040231,0.));
#12992=DIRECTION('center_axis',(0.,0.,1.));
#12993=DIRECTION('ref_axis',(1.,0.,0.));
#12994=DIRECTION('',(0.156434465040224,0.987688340595139,0.));
#12995=DIRECTION('center_axis',(0.,0.,1.));
#12996=DIRECTION('ref_axis',(1.,0.,0.));
#12997=DIRECTION('',(0.156434465040224,0.987688340595139,0.));
#12998=DIRECTION('center_axis',(-0.987688340595139,0.156434465040224,0.));
#12999=DIRECTION('ref_axis',(-0.156434465040224,-0.987688340595139,0.));
#13000=DIRECTION('center_axis',(-0.309016994374948,-0.951056516295154,0.));
#13001=DIRECTION('ref_axis',(0.951056516295154,-0.309016994374948,0.));
#13002=DIRECTION('',(-0.951056516295153,0.309016994374948,0.));
#13003=DIRECTION('',(0.,0.,-1.));
#13004=DIRECTION('',(-0.951056516295153,0.309016994374948,0.));
#13005=DIRECTION('center_axis',(0.309016994374947,0.951056516295154,0.));
#13006=DIRECTION('ref_axis',(-0.951056516295154,0.309016994374947,0.));
#13007=DIRECTION('',(0.951056516295154,-0.309016994374947,0.));
#13008=DIRECTION('',(0.,0.,-1.));
#13009=DIRECTION('',(0.951056516295154,-0.309016994374947,0.));
#13010=DIRECTION('center_axis',(0.,0.,1.));
#13011=DIRECTION('ref_axis',(1.,0.,0.));
#13012=DIRECTION('',(0.309016994374941,0.951056516295156,0.));
#13013=DIRECTION('center_axis',(0.,0.,1.));
#13014=DIRECTION('ref_axis',(1.,0.,0.));
#13015=DIRECTION('',(0.309016994374941,0.951056516295156,0.));
#13016=DIRECTION('center_axis',(-0.951056516295156,0.309016994374941,0.));
#13017=DIRECTION('ref_axis',(-0.309016994374941,-0.951056516295156,0.));
#13018=DIRECTION('center_axis',(-0.453990499739548,-0.891006524188367,0.));
#13019=DIRECTION('ref_axis',(0.891006524188367,-0.453990499739548,0.));
#13020=DIRECTION('',(-0.891006524188367,0.453990499739548,0.));
#13021=DIRECTION('',(0.,0.,-1.));
#13022=DIRECTION('',(-0.891006524188367,0.453990499739548,0.));
#13023=DIRECTION('center_axis',(0.453990499739548,0.891006524188367,0.));
#13024=DIRECTION('ref_axis',(-0.891006524188367,0.453990499739548,0.));
#13025=DIRECTION('',(0.891006524188367,-0.453990499739548,0.));
#13026=DIRECTION('',(0.,0.,-1.));
#13027=DIRECTION('',(0.891006524188367,-0.453990499739548,0.));
#13028=DIRECTION('center_axis',(0.,0.,1.));
#13029=DIRECTION('ref_axis',(1.,0.,0.));
#13030=DIRECTION('',(0.453990499739554,0.891006524188364,0.));
#13031=DIRECTION('center_axis',(0.,0.,1.));
#13032=DIRECTION('ref_axis',(1.,0.,0.));
#13033=DIRECTION('',(0.453990499739554,0.891006524188364,0.));
#13034=DIRECTION('center_axis',(-0.891006524188364,0.453990499739554,0.));
#13035=DIRECTION('ref_axis',(-0.453990499739554,-0.891006524188364,0.));
#13036=DIRECTION('center_axis',(-0.587785252292473,-0.809016994374947,0.));
#13037=DIRECTION('ref_axis',(0.809016994374947,-0.587785252292473,0.));
#13038=DIRECTION('',(-0.809016994374947,0.587785252292473,0.));
#13039=DIRECTION('',(0.,0.,-1.));
#13040=DIRECTION('',(-0.809016994374947,0.587785252292473,0.));
#13041=DIRECTION('center_axis',(0.587785252292474,0.809016994374946,0.));
#13042=DIRECTION('ref_axis',(-0.809016994374946,0.587785252292474,0.));
#13043=DIRECTION('',(0.809016994374946,-0.587785252292474,0.));
#13044=DIRECTION('',(0.,0.,-1.));
#13045=DIRECTION('',(0.809016994374946,-0.587785252292474,0.));
#13046=DIRECTION('center_axis',(0.,0.,1.));
#13047=DIRECTION('ref_axis',(1.,0.,0.));
#13048=DIRECTION('',(0.587785252292475,0.809016994374946,0.));
#13049=DIRECTION('center_axis',(0.,0.,1.));
#13050=DIRECTION('ref_axis',(1.,0.,0.));
#13051=DIRECTION('',(0.587785252292475,0.809016994374946,0.));
#13052=DIRECTION('center_axis',(-0.809016994374946,0.587785252292475,0.));
#13053=DIRECTION('ref_axis',(-0.587785252292475,-0.809016994374946,0.));
#13054=DIRECTION('center_axis',(-0.809016994374948,-0.587785252292472,0.));
#13055=DIRECTION('ref_axis',(0.587785252292472,-0.809016994374948,0.));
#13056=DIRECTION('',(-0.587785252292472,0.809016994374948,0.));
#13057=DIRECTION('',(0.,0.,-1.));
#13058=DIRECTION('',(-0.587785252292472,0.809016994374948,0.));
#13059=DIRECTION('center_axis',(0.809016994374948,0.587785252292472,0.));
#13060=DIRECTION('ref_axis',(-0.587785252292472,0.809016994374948,0.));
#13061=DIRECTION('',(0.587785252292472,-0.809016994374948,0.));
#13062=DIRECTION('',(0.,0.,-1.));
#13063=DIRECTION('',(0.587785252292472,-0.809016994374948,0.));
#13064=DIRECTION('center_axis',(0.,0.,1.));
#13065=DIRECTION('ref_axis',(1.,0.,0.));
#13066=DIRECTION('',(0.809016994374946,0.587785252292475,0.));
#13067=DIRECTION('center_axis',(0.,0.,1.));
#13068=DIRECTION('ref_axis',(1.,0.,0.));
#13069=DIRECTION('',(0.809016994374946,0.587785252292475,0.));
#13070=DIRECTION('center_axis',(-0.587785252292475,0.809016994374946,0.));
#13071=DIRECTION('ref_axis',(-0.809016994374946,-0.587785252292475,0.));
#13072=DIRECTION('center_axis',(-0.891006524188367,-0.453990499739548,0.));
#13073=DIRECTION('ref_axis',(0.453990499739548,-0.891006524188367,0.));
#13074=DIRECTION('',(-0.453990499739548,0.891006524188367,0.));
#13075=DIRECTION('',(0.,0.,-1.));
#13076=DIRECTION('',(-0.453990499739548,0.891006524188367,0.));
#13077=DIRECTION('center_axis',(0.891006524188367,0.453990499739548,0.));
#13078=DIRECTION('ref_axis',(-0.453990499739548,0.891006524188367,0.));
#13079=DIRECTION('',(0.453990499739548,-0.891006524188367,0.));
#13080=DIRECTION('',(0.,0.,-1.));
#13081=DIRECTION('',(0.453990499739548,-0.891006524188367,0.));
#13082=DIRECTION('center_axis',(0.,0.,1.));
#13083=DIRECTION('ref_axis',(1.,0.,0.));
#13084=DIRECTION('',(0.891006524188364,0.453990499739554,0.));
#13085=DIRECTION('center_axis',(0.,0.,1.));
#13086=DIRECTION('ref_axis',(1.,0.,0.));
#13087=DIRECTION('',(0.891006524188364,0.453990499739554,0.));
#13088=DIRECTION('center_axis',(-0.453990499739554,0.891006524188364,0.));
#13089=DIRECTION('ref_axis',(-0.891006524188364,-0.453990499739554,0.));
#13090=DIRECTION('center_axis',(-0.951056516295154,-0.309016994374947,0.));
#13091=DIRECTION('ref_axis',(0.309016994374947,-0.951056516295154,0.));
#13092=DIRECTION('',(-0.309016994374947,0.951056516295154,0.));
#13093=DIRECTION('',(0.,0.,-1.));
#13094=DIRECTION('',(-0.309016994374947,0.951056516295154,0.));
#13095=DIRECTION('center_axis',(0.951056516295154,0.309016994374947,0.));
#13096=DIRECTION('ref_axis',(-0.309016994374947,0.951056516295154,0.));
#13097=DIRECTION('',(0.309016994374947,-0.951056516295154,0.));
#13098=DIRECTION('',(0.,0.,-1.));
#13099=DIRECTION('',(0.309016994374947,-0.951056516295154,0.));
#13100=DIRECTION('center_axis',(0.,0.,1.));
#13101=DIRECTION('ref_axis',(1.,0.,0.));
#13102=DIRECTION('',(0.951056516295156,0.309016994374941,0.));
#13103=DIRECTION('center_axis',(0.,0.,1.));
#13104=DIRECTION('ref_axis',(1.,0.,0.));
#13105=DIRECTION('',(0.951056516295156,0.309016994374941,0.));
#13106=DIRECTION('center_axis',(-0.309016994374941,0.951056516295156,0.));
#13107=DIRECTION('ref_axis',(-0.951056516295156,-0.309016994374941,0.));
#13108=DIRECTION('center_axis',(-0.987688340595138,-0.156434465040231,0.));
#13109=DIRECTION('ref_axis',(0.156434465040231,-0.987688340595138,0.));
#13110=DIRECTION('',(-0.156434465040231,0.987688340595138,0.));
#13111=DIRECTION('',(0.,0.,-1.));
#13112=DIRECTION('',(-0.156434465040231,0.987688340595138,0.));
#13113=DIRECTION('center_axis',(0.987688340595138,0.156434465040231,0.));
#13114=DIRECTION('ref_axis',(-0.156434465040231,0.987688340595138,0.));
#13115=DIRECTION('',(0.156434465040231,-0.987688340595138,0.));
#13116=DIRECTION('',(0.,0.,-1.));
#13117=DIRECTION('',(0.156434465040231,-0.987688340595138,0.));
#13118=DIRECTION('center_axis',(0.,0.,1.));
#13119=DIRECTION('ref_axis',(1.,0.,0.));
#13120=DIRECTION('',(0.987688340595139,0.156434465040223,0.));
#13121=DIRECTION('center_axis',(0.,0.,1.));
#13122=DIRECTION('ref_axis',(1.,0.,0.));
#13123=DIRECTION('',(0.987688340595139,0.156434465040223,0.));
#13124=DIRECTION('center_axis',(-0.156434465040223,0.987688340595139,0.));
#13125=DIRECTION('ref_axis',(-0.987688340595139,-0.156434465040223,0.));
#13126=DIRECTION('center_axis',(-0.987688340595138,0.156434465040231,0.));
#13127=DIRECTION('ref_axis',(-0.156434465040231,-0.987688340595138,0.));
#13128=DIRECTION('',(0.156434465040231,0.987688340595138,0.));
#13129=DIRECTION('',(0.,0.,-1.));
#13130=DIRECTION('',(0.156434465040231,0.987688340595138,0.));
#13131=DIRECTION('center_axis',(0.987688340595138,-0.156434465040232,0.));
#13132=DIRECTION('ref_axis',(0.156434465040232,0.987688340595138,0.));
#13133=DIRECTION('',(-0.156434465040232,-0.987688340595138,0.));
#13134=DIRECTION('',(0.,0.,-1.));
#13135=DIRECTION('',(-0.156434465040232,-0.987688340595138,0.));
#13136=DIRECTION('center_axis',(0.,0.,1.));
#13137=DIRECTION('ref_axis',(1.,0.,0.));
#13138=DIRECTION('',(0.987688340595139,-0.156434465040223,0.));
#13139=DIRECTION('center_axis',(0.,0.,1.));
#13140=DIRECTION('ref_axis',(1.,0.,0.));
#13141=DIRECTION('',(0.987688340595139,-0.156434465040223,0.));
#13142=DIRECTION('center_axis',(0.156434465040223,0.987688340595139,0.));
#13143=DIRECTION('ref_axis',(-0.987688340595139,0.156434465040223,0.));
#13144=DIRECTION('center_axis',(-0.951056516295154,0.309016994374948,0.));
#13145=DIRECTION('ref_axis',(-0.309016994374948,-0.951056516295154,0.));
#13146=DIRECTION('',(0.309016994374948,0.951056516295153,0.));
#13147=DIRECTION('',(0.,0.,-1.));
#13148=DIRECTION('',(0.309016994374948,0.951056516295153,0.));
#13149=DIRECTION('center_axis',(0.951056516295154,-0.309016994374947,0.));
#13150=DIRECTION('ref_axis',(0.309016994374947,0.951056516295154,0.));
#13151=DIRECTION('',(-0.309016994374947,-0.951056516295154,0.));
#13152=DIRECTION('',(0.,0.,-1.));
#13153=DIRECTION('',(-0.309016994374947,-0.951056516295154,0.));
#13154=DIRECTION('center_axis',(0.,0.,1.));
#13155=DIRECTION('ref_axis',(1.,0.,0.));
#13156=DIRECTION('',(0.951056516295156,-0.309016994374941,0.));
#13157=DIRECTION('center_axis',(0.,0.,1.));
#13158=DIRECTION('ref_axis',(1.,0.,0.));
#13159=DIRECTION('',(0.951056516295156,-0.309016994374941,0.));
#13160=DIRECTION('center_axis',(0.309016994374941,0.951056516295156,0.));
#13161=DIRECTION('ref_axis',(-0.951056516295156,0.309016994374941,0.));
#13162=DIRECTION('center_axis',(-0.891006524188367,0.453990499739548,0.));
#13163=DIRECTION('ref_axis',(-0.453990499739548,-0.891006524188367,0.));
#13164=DIRECTION('',(0.453990499739548,0.891006524188367,0.));
#13165=DIRECTION('',(0.,0.,-1.));
#13166=DIRECTION('',(0.453990499739548,0.891006524188367,0.));
#13167=DIRECTION('center_axis',(0.891006524188367,-0.453990499739548,0.));
#13168=DIRECTION('ref_axis',(0.453990499739548,0.891006524188367,0.));
#13169=DIRECTION('',(-0.453990499739548,-0.891006524188367,0.));
#13170=DIRECTION('',(0.,0.,-1.));
#13171=DIRECTION('',(-0.453990499739548,-0.891006524188367,0.));
#13172=DIRECTION('center_axis',(0.,0.,1.));
#13173=DIRECTION('ref_axis',(1.,0.,0.));
#13174=DIRECTION('',(0.891006524188364,-0.453990499739554,0.));
#13175=DIRECTION('center_axis',(0.,0.,1.));
#13176=DIRECTION('ref_axis',(1.,0.,0.));
#13177=DIRECTION('',(0.891006524188364,-0.453990499739554,0.));
#13178=DIRECTION('center_axis',(0.453990499739554,0.891006524188364,0.));
#13179=DIRECTION('ref_axis',(-0.891006524188364,0.453990499739554,0.));
#13180=DIRECTION('center_axis',(-0.809016994374948,0.587785252292472,0.));
#13181=DIRECTION('ref_axis',(-0.587785252292472,-0.809016994374948,0.));
#13182=DIRECTION('',(0.587785252292472,0.809016994374948,0.));
#13183=DIRECTION('',(0.,0.,-1.));
#13184=DIRECTION('',(0.587785252292472,0.809016994374948,0.));
#13185=DIRECTION('center_axis',(0.809016994374948,-0.587785252292472,0.));
#13186=DIRECTION('ref_axis',(0.587785252292472,0.809016994374948,0.));
#13187=DIRECTION('',(-0.587785252292472,-0.809016994374948,0.));
#13188=DIRECTION('',(0.,0.,-1.));
#13189=DIRECTION('',(-0.587785252292472,-0.809016994374948,0.));
#13190=DIRECTION('center_axis',(0.,0.,1.));
#13191=DIRECTION('ref_axis',(1.,0.,0.));
#13192=DIRECTION('',(0.809016994374946,-0.587785252292475,0.));
#13193=DIRECTION('center_axis',(0.,0.,1.));
#13194=DIRECTION('ref_axis',(1.,0.,0.));
#13195=DIRECTION('',(0.809016994374946,-0.587785252292475,0.));
#13196=DIRECTION('center_axis',(0.587785252292475,0.809016994374946,0.));
#13197=DIRECTION('ref_axis',(-0.809016994374946,0.587785252292475,0.));
#13198=DIRECTION('center_axis',(-0.587785252292472,0.809016994374948,0.));
#13199=DIRECTION('ref_axis',(-0.809016994374948,-0.587785252292472,0.));
#13200=DIRECTION('',(0.809016994374948,0.587785252292472,0.));
#13201=DIRECTION('',(0.,0.,-1.));
#13202=DIRECTION('',(0.809016994374948,0.587785252292472,0.));
#13203=DIRECTION('center_axis',(0.587785252292472,-0.809016994374948,0.));
#13204=DIRECTION('ref_axis',(0.809016994374948,0.587785252292472,0.));
#13205=DIRECTION('',(-0.809016994374948,-0.587785252292472,0.));
#13206=DIRECTION('',(0.,0.,-1.));
#13207=DIRECTION('',(-0.809016994374948,-0.587785252292472,0.));
#13208=DIRECTION('center_axis',(0.,0.,1.));
#13209=DIRECTION('ref_axis',(1.,0.,0.));
#13210=DIRECTION('',(0.587785252292475,-0.809016994374946,0.));
#13211=DIRECTION('center_axis',(0.,0.,1.));
#13212=DIRECTION('ref_axis',(1.,0.,0.));
#13213=DIRECTION('',(0.587785252292475,-0.809016994374946,0.));
#13214=DIRECTION('center_axis',(0.809016994374946,0.587785252292475,0.));
#13215=DIRECTION('ref_axis',(-0.587785252292475,0.809016994374946,0.));
#13216=DIRECTION('center_axis',(-0.453990499739548,0.891006524188367,0.));
#13217=DIRECTION('ref_axis',(-0.891006524188367,-0.453990499739548,0.));
#13218=DIRECTION('',(0.891006524188367,0.453990499739548,0.));
#13219=DIRECTION('',(0.,0.,-1.));
#13220=DIRECTION('',(0.891006524188367,0.453990499739548,0.));
#13221=DIRECTION('center_axis',(0.453990499739548,-0.891006524188367,0.));
#13222=DIRECTION('ref_axis',(0.891006524188367,0.453990499739548,0.));
#13223=DIRECTION('',(-0.891006524188367,-0.453990499739548,0.));
#13224=DIRECTION('',(0.,0.,-1.));
#13225=DIRECTION('',(-0.891006524188367,-0.453990499739548,0.));
#13226=DIRECTION('center_axis',(0.,0.,1.));
#13227=DIRECTION('ref_axis',(1.,0.,0.));
#13228=DIRECTION('',(0.453990499739554,-0.891006524188364,0.));
#13229=DIRECTION('center_axis',(0.,0.,1.));
#13230=DIRECTION('ref_axis',(1.,0.,0.));
#13231=DIRECTION('',(0.453990499739554,-0.891006524188364,0.));
#13232=DIRECTION('center_axis',(0.891006524188364,0.453990499739554,0.));
#13233=DIRECTION('ref_axis',(-0.453990499739554,0.891006524188364,0.));
#13234=DIRECTION('center_axis',(-0.309016994374947,0.951056516295154,0.));
#13235=DIRECTION('ref_axis',(-0.951056516295154,-0.309016994374947,0.));
#13236=DIRECTION('',(0.951056516295154,0.309016994374947,0.));
#13237=DIRECTION('',(0.,0.,-1.));
#13238=DIRECTION('',(0.951056516295154,0.309016994374947,0.));
#13239=DIRECTION('center_axis',(0.309016994374948,-0.951056516295154,0.));
#13240=DIRECTION('ref_axis',(0.951056516295154,0.309016994374948,0.));
#13241=DIRECTION('',(-0.951056516295153,-0.309016994374948,0.));
#13242=DIRECTION('',(0.,0.,-1.));
#13243=DIRECTION('',(-0.951056516295153,-0.309016994374948,0.));
#13244=DIRECTION('center_axis',(0.,0.,1.));
#13245=DIRECTION('ref_axis',(1.,0.,0.));
#13246=DIRECTION('',(0.309016994374941,-0.951056516295156,0.));
#13247=DIRECTION('center_axis',(0.,0.,1.));
#13248=DIRECTION('ref_axis',(1.,0.,0.));
#13249=DIRECTION('',(0.309016994374941,-0.951056516295156,0.));
#13250=DIRECTION('center_axis',(0.951056516295156,0.309016994374941,0.));
#13251=DIRECTION('ref_axis',(-0.309016994374941,0.951056516295156,0.));
#15146=CARTESIAN_POINT('',(0.,0.,0.));
#15147=CARTESIAN_POINT('Origin',(0.,0.,22.));
#15148=CARTESIAN_POINT('',(6.2,-7.59281015471359E-16,22.));
#15149=CARTESIAN_POINT('Origin',(0.,0.,22.));
#15150=CARTESIAN_POINT('',(6.2,-7.59281015471359E-16,0.));
#15151=CARTESIAN_POINT('',(6.2,-7.59281015471359E-16,22.));
#15152=CARTESIAN_POINT('Origin',(0.,0.,0.));
#15153=CARTESIAN_POINT('Origin',(0.,0.,22.));
#15154=CARTESIAN_POINT('',(14.,-1.71450551880629E-15,0.));
#15155=CARTESIAN_POINT('Origin',(0.,0.,0.));
#15156=CARTESIAN_POINT('',(14.,-1.71450551880629E-15,1.));
#15157=CARTESIAN_POINT('',(14.,-1.71450551880629E-15,22.));
#15158=CARTESIAN_POINT('',(13.9994857048393,-0.12,1.));
#15159=CARTESIAN_POINT('Origin',(0.,0.,1.));
#15160=CARTESIAN_POINT('',(13.9994857048393,-0.12,7.));
#15161=CARTESIAN_POINT('',(13.9994857048393,-0.12,22.));
#15162=CARTESIAN_POINT('',(14.,-1.71450551880629E-15,7.));
#15163=CARTESIAN_POINT('Origin',(0.,0.,7.));
#15164=CARTESIAN_POINT('',(14.,-1.71450551880629E-15,22.));
#15165=CARTESIAN_POINT('',(14.,-1.71450551880629E-15,22.));
#15166=CARTESIAN_POINT('Origin',(0.,0.,22.));
#15167=CARTESIAN_POINT('',(13.9994857048393,0.12,7.));
#15168=CARTESIAN_POINT('Origin',(0.,0.,7.));
#15169=CARTESIAN_POINT('',(13.9994857048393,0.12,1.));
#15170=CARTESIAN_POINT('',(13.9994857048393,0.12,22.));
#15171=CARTESIAN_POINT('Origin',(0.,0.,1.));
#15172=CARTESIAN_POINT('',(-13.9994857048393,0.120000000000002,7.));
#15173=CARTESIAN_POINT('',(-13.9994857048393,-0.119999999999998,7.));
#15174=CARTESIAN_POINT('Origin',(0.,0.,7.));
#15175=CARTESIAN_POINT('',(-13.9994857048393,-0.119999999999998,1.));
#15176=CARTESIAN_POINT('',(-13.9994857048393,-0.119999999999998,22.));
#15177=CARTESIAN_POINT('',(-13.9994857048393,0.120000000000002,1.));
#15178=CARTESIAN_POINT('Origin',(0.,0.,1.));
#15179=CARTESIAN_POINT('',(-13.9994857048393,0.120000000000002,22.));
#15180=CARTESIAN_POINT('',(9.81427846127362,-9.98398408875839,7.));
#15181=CARTESIAN_POINT('',(9.81427846127362,-9.98398408875839,1.));
#15182=CARTESIAN_POINT('',(9.81427846127362,-9.98398408875839,22.));
#15183=CARTESIAN_POINT('',(9.98398408875839,-9.81427846127362,7.));
#15184=CARTESIAN_POINT('Origin',(0.,0.,7.));
#15185=CARTESIAN_POINT('',(9.98398408875839,-9.81427846127362,1.));
#15186=CARTESIAN_POINT('',(9.98398408875839,-9.81427846127362,22.));
#15187=CARTESIAN_POINT('Origin',(0.,0.,1.));
#15188=CARTESIAN_POINT('',(-0.120000000000003,-13.9994857048393,7.));
#15189=CARTESIAN_POINT('',(-0.120000000000003,-13.9994857048393,1.));
#15190=CARTESIAN_POINT('',(-0.120000000000003,-13.9994857048393,22.));
#15191=CARTESIAN_POINT('',(0.119999999999997,-13.9994857048393,7.));
#15192=CARTESIAN_POINT('Origin',(0.,0.,7.));
#15193=CARTESIAN_POINT('',(0.119999999999997,-13.9994857048393,1.));
#15194=CARTESIAN_POINT('',(0.119999999999997,-13.9994857048393,22.));
#15195=CARTESIAN_POINT('Origin',(0.,0.,1.));
#15196=CARTESIAN_POINT('',(-9.98398408875839,-9.81427846127362,7.));
#15197=CARTESIAN_POINT('',(-9.98398408875839,-9.81427846127362,1.));
#15198=CARTESIAN_POINT('',(-9.98398408875839,-9.81427846127362,22.));
#15199=CARTESIAN_POINT('',(-9.81427846127362,-9.98398408875839,7.));
#15200=CARTESIAN_POINT('Origin',(0.,0.,7.));
#15201=CARTESIAN_POINT('',(-9.81427846127362,-9.98398408875839,1.));
#15202=CARTESIAN_POINT('',(-9.81427846127362,-9.98398408875839,22.));
#15203=CARTESIAN_POINT('Origin',(0.,0.,1.));
#15204=CARTESIAN_POINT('',(13.8083566691933,-2.30852465794632,4.));
#15205=CARTESIAN_POINT('',(13.8083566691933,-2.30852465794632,1.));
#15206=CARTESIAN_POINT('',(13.8083566691933,-2.30852465794632,22.));
#15207=CARTESIAN_POINT('',(13.8459009408029,-2.07147945620348,4.));
#15208=CARTESIAN_POINT('Origin',(0.,0.,4.));
#15209=CARTESIAN_POINT('',(13.8459009408029,-2.07147945620348,1.));
#15210=CARTESIAN_POINT('',(13.8459009408029,-2.07147945620348,22.));
#15211=CARTESIAN_POINT('Origin',(0.,0.,1.));
#15212=CARTESIAN_POINT('',(13.2772200650433,-4.44020577725991,4.));
#15213=CARTESIAN_POINT('',(13.2772200650433,-4.44020577725991,1.));
#15214=CARTESIAN_POINT('',(13.2772200650433,-4.44020577725991,22.));
#15215=CARTESIAN_POINT('',(13.3513841436933,-4.21195221334907,4.));
#15216=CARTESIAN_POINT('Origin',(0.,0.,4.));
#15217=CARTESIAN_POINT('',(13.3513841436933,-4.21195221334907,1.));
#15218=CARTESIAN_POINT('',(13.3513841436933,-4.21195221334907,22.));
#15219=CARTESIAN_POINT('Origin',(0.,0.,1.));
#15220=CARTESIAN_POINT('',(12.4191542383249,-6.46255429413924,4.));
#15221=CARTESIAN_POINT('',(12.4191542383249,-6.46255429413924,1.));
#15222=CARTESIAN_POINT('',(12.4191542383249,-6.46255429413924,22.));
#15223=CARTESIAN_POINT('',(12.5281119582624,-6.24871272833404,4.));
#15224=CARTESIAN_POINT('Origin',(0.,0.,4.));
#15225=CARTESIAN_POINT('',(12.5281119582624,-6.24871272833404,1.));
#15226=CARTESIAN_POINT('',(12.5281119582624,-6.24871272833404,22.));
#15227=CARTESIAN_POINT('Origin',(0.,0.,1.));
#15228=CARTESIAN_POINT('',(11.255287617449,-8.32577327630884,4.));
#15229=CARTESIAN_POINT('',(11.255287617449,-8.32577327630884,1.));
#15230=CARTESIAN_POINT('',(11.255287617449,-8.32577327630884,22.));
#15231=CARTESIAN_POINT('',(11.3963560779992,-8.13160919765885,4.));
#15232=CARTESIAN_POINT('Origin',(0.,0.,4.));
#15233=CARTESIAN_POINT('',(11.3963560779992,-8.13160919765885,1.));
#15234=CARTESIAN_POINT('',(11.3963560779992,-8.13160919765885,22.));
#15235=CARTESIAN_POINT('Origin',(0.,0.,1.));
#15236=CARTESIAN_POINT('',(8.13160919765884,-11.3963560779992,4.));
#15237=CARTESIAN_POINT('',(8.13160919765884,-11.3963560779992,1.));
#15238=CARTESIAN_POINT('',(8.13160919765884,-11.3963560779992,22.));
#15239=CARTESIAN_POINT('',(8.32577327630883,-11.255287617449,4.));
#15240=CARTESIAN_POINT('Origin',(0.,0.,4.));
#15241=CARTESIAN_POINT('',(8.32577327630883,-11.255287617449,1.));
#15242=CARTESIAN_POINT('',(8.32577327630883,-11.255287617449,22.));
#15243=CARTESIAN_POINT('Origin',(0.,0.,1.));
#15244=CARTESIAN_POINT('',(6.24871272833403,-12.5281119582624,4.));
#15245=CARTESIAN_POINT('',(6.24871272833403,-12.5281119582624,1.));
#15246=CARTESIAN_POINT('',(6.24871272833403,-12.5281119582624,22.));
#15247=CARTESIAN_POINT('',(6.46255429413924,-12.4191542383249,4.));
#15248=CARTESIAN_POINT('Origin',(0.,0.,4.));
#15249=CARTESIAN_POINT('',(6.46255429413924,-12.4191542383249,1.));
#15250=CARTESIAN_POINT('',(6.46255429413924,-12.4191542383249,22.));
#15251=CARTESIAN_POINT('Origin',(0.,0.,1.));
#15252=CARTESIAN_POINT('',(4.21195221334906,-13.3513841436933,4.));
#15253=CARTESIAN_POINT('',(4.21195221334906,-13.3513841436933,1.));
#15254=CARTESIAN_POINT('',(4.21195221334906,-13.3513841436933,22.));
#15255=CARTESIAN_POINT('',(4.4402057772599,-13.2772200650433,4.));
#15256=CARTESIAN_POINT('Origin',(0.,0.,4.));
#15257=CARTESIAN_POINT('',(4.4402057772599,-13.2772200650433,1.));
#15258=CARTESIAN_POINT('',(4.4402057772599,-13.2772200650433,22.));
#15259=CARTESIAN_POINT('Origin',(0.,0.,1.));
#15260=CARTESIAN_POINT('',(2.07147945620348,-13.8459009408029,4.));
#15261=CARTESIAN_POINT('',(2.07147945620348,-13.8459009408029,1.));
#15262=CARTESIAN_POINT('',(2.07147945620348,-13.8459009408029,22.));
#15263=CARTESIAN_POINT('',(2.30852465794631,-13.8083566691933,4.));
#15264=CARTESIAN_POINT('Origin',(0.,0.,4.));
#15265=CARTESIAN_POINT('',(2.30852465794631,-13.8083566691933,1.));
#15266=CARTESIAN_POINT('',(2.30852465794631,-13.8083566691933,22.));
#15267=CARTESIAN_POINT('Origin',(0.,0.,1.));
#15268=CARTESIAN_POINT('',(-2.30852465794632,-13.8083566691933,4.));
#15269=CARTESIAN_POINT('',(-2.30852465794632,-13.8083566691933,1.));
#15270=CARTESIAN_POINT('',(-2.30852465794631,-13.8083566691933,22.));
#15271=CARTESIAN_POINT('',(-2.07147945620348,-13.8459009408029,4.));
#15272=CARTESIAN_POINT('Origin',(0.,0.,4.));
#15273=CARTESIAN_POINT('',(-2.07147945620348,-13.8459009408029,1.));
#15274=CARTESIAN_POINT('',(-2.07147945620348,-13.8459009408029,22.));
#15275=CARTESIAN_POINT('Origin',(0.,0.,1.));
#15276=CARTESIAN_POINT('',(-4.44020577725991,-13.2772200650433,4.));
#15277=CARTESIAN_POINT('',(-4.44020577725991,-13.2772200650433,1.));
#15278=CARTESIAN_POINT('',(-4.4402057772599,-13.2772200650433,22.));
#15279=CARTESIAN_POINT('',(-4.21195221334907,-13.3513841436933,4.));
#15280=CARTESIAN_POINT('Origin',(0.,0.,4.));
#15281=CARTESIAN_POINT('',(-4.21195221334907,-13.3513841436933,1.));
#15282=CARTESIAN_POINT('',(-4.21195221334907,-13.3513841436933,22.));
#15283=CARTESIAN_POINT('Origin',(0.,0.,1.));
#15284=CARTESIAN_POINT('',(-6.46255429413924,-12.4191542383249,4.));
#15285=CARTESIAN_POINT('',(-6.46255429413924,-12.4191542383249,1.));
#15286=CARTESIAN_POINT('',(-6.46255429413924,-12.4191542383249,22.));
#15287=CARTESIAN_POINT('',(-6.24871272833404,-12.5281119582624,4.));
#15288=CARTESIAN_POINT('Origin',(0.,0.,4.));
#15289=CARTESIAN_POINT('',(-6.24871272833404,-12.5281119582624,1.));
#15290=CARTESIAN_POINT('',(-6.24871272833404,-12.5281119582624,22.));
#15291=CARTESIAN_POINT('Origin',(0.,0.,1.));
#15292=CARTESIAN_POINT('',(-8.32577327630884,-11.255287617449,4.));
#15293=CARTESIAN_POINT('',(-8.32577327630884,-11.255287617449,1.));
#15294=CARTESIAN_POINT('',(-8.32577327630884,-11.255287617449,22.));
#15295=CARTESIAN_POINT('',(-8.13160919765885,-11.3963560779992,4.));
#15296=CARTESIAN_POINT('Origin',(0.,0.,4.));
#15297=CARTESIAN_POINT('',(-8.13160919765885,-11.3963560779992,1.));
#15298=CARTESIAN_POINT('',(-8.13160919765885,-11.3963560779992,22.));
#15299=CARTESIAN_POINT('Origin',(0.,0.,1.));
#15300=CARTESIAN_POINT('',(-11.3963560779992,-8.13160919765885,4.));
#15301=CARTESIAN_POINT('',(-11.3963560779992,-8.13160919765885,1.));
#15302=CARTESIAN_POINT('',(-11.3963560779992,-8.13160919765885,22.));
#15303=CARTESIAN_POINT('',(-11.255287617449,-8.32577327630884,4.));
#15304=CARTESIAN_POINT('Origin',(0.,0.,4.));
#15305=CARTESIAN_POINT('',(-11.255287617449,-8.32577327630884,1.));
#15306=CARTESIAN_POINT('',(-11.255287617449,-8.32577327630884,22.));
#15307=CARTESIAN_POINT('Origin',(0.,0.,1.));
#15308=CARTESIAN_POINT('',(-12.5281119582624,-6.24871272833403,4.));
#15309=CARTESIAN_POINT('',(-12.5281119582624,-6.24871272833403,1.));
#15310=CARTESIAN_POINT('',(-12.5281119582624,-6.24871272833403,22.));
#15311=CARTESIAN_POINT('',(-12.4191542383249,-6.46255429413924,4.));
#15312=CARTESIAN_POINT('Origin',(0.,0.,4.));
#15313=CARTESIAN_POINT('',(-12.4191542383249,-6.46255429413924,1.));
#15314=CARTESIAN_POINT('',(-12.4191542383249,-6.46255429413924,22.));
#15315=CARTESIAN_POINT('Origin',(0.,0.,1.));
#15316=CARTESIAN_POINT('',(-13.3513841436933,-4.21195221334906,4.));
#15317=CARTESIAN_POINT('',(-13.3513841436933,-4.21195221334906,1.));
#15318=CARTESIAN_POINT('',(-13.3513841436933,-4.21195221334906,22.));
#15319=CARTESIAN_POINT('',(-13.2772200650433,-4.44020577725989,4.));
#15320=CARTESIAN_POINT('Origin',(0.,0.,4.));
#15321=CARTESIAN_POINT('',(-13.2772200650433,-4.44020577725989,1.));
#15322=CARTESIAN_POINT('',(-13.2772200650433,-4.44020577725989,22.));
#15323=CARTESIAN_POINT('Origin',(0.,0.,1.));
#15324=CARTESIAN_POINT('',(-13.8459009408029,-2.07147945620348,4.));
#15325=CARTESIAN_POINT('',(-13.8459009408029,-2.07147945620348,1.));
#15326=CARTESIAN_POINT('',(-13.8459009408029,-2.07147945620348,22.));
#15327=CARTESIAN_POINT('',(-13.8083566691933,-2.30852465794631,4.));
#15328=CARTESIAN_POINT('Origin',(0.,0.,4.));
#15329=CARTESIAN_POINT('',(-13.8083566691933,-2.30852465794631,1.));
#15330=CARTESIAN_POINT('',(-13.8083566691933,-2.30852465794631,22.));
#15331=CARTESIAN_POINT('Origin',(0.,0.,1.));
#15332=CARTESIAN_POINT('',(-9.81427846127362,9.98398408875839,7.));
#15333=CARTESIAN_POINT('',(-9.81427846127362,9.98398408875839,1.));
#15334=CARTESIAN_POINT('',(-9.81427846127362,9.98398408875839,22.));
#15335=CARTESIAN_POINT('',(-9.98398408875839,9.81427846127362,7.));
#15336=CARTESIAN_POINT('Origin',(0.,0.,7.));
#15337=CARTESIAN_POINT('',(-9.98398408875839,9.81427846127362,1.));
#15338=CARTESIAN_POINT('',(-9.98398408875839,9.81427846127362,22.));
#15339=CARTESIAN_POINT('Origin',(0.,0.,1.));
#15340=CARTESIAN_POINT('',(0.120000000000001,13.9994857048393,7.));
#15341=CARTESIAN_POINT('',(0.120000000000001,13.9994857048393,1.));
#15342=CARTESIAN_POINT('',(0.120000000000001,13.9994857048393,22.));
#15343=CARTESIAN_POINT('',(-0.119999999999999,13.9994857048393,7.));
#15344=CARTESIAN_POINT('Origin',(0.,0.,7.));
#15345=CARTESIAN_POINT('',(-0.119999999999999,13.9994857048393,1.));
#15346=CARTESIAN_POINT('',(-0.119999999999999,13.9994857048393,22.));
#15347=CARTESIAN_POINT('Origin',(0.,0.,1.));
#15348=CARTESIAN_POINT('',(9.98398408875839,9.81427846127362,7.));
#15349=CARTESIAN_POINT('',(9.98398408875839,9.81427846127362,1.));
#15350=CARTESIAN_POINT('',(9.98398408875839,9.81427846127362,22.));
#15351=CARTESIAN_POINT('',(9.81427846127362,9.98398408875839,7.));
#15352=CARTESIAN_POINT('Origin',(0.,0.,7.));
#15353=CARTESIAN_POINT('',(9.81427846127362,9.98398408875839,1.));
#15354=CARTESIAN_POINT('',(9.81427846127362,9.98398408875839,22.));
#15355=CARTESIAN_POINT('Origin',(0.,0.,1.));
#15356=CARTESIAN_POINT('',(13.8459009408029,2.07147945620348,4.));
#15357=CARTESIAN_POINT('',(13.8459009408029,2.07147945620348,1.));
#15358=CARTESIAN_POINT('',(13.8459009408029,2.07147945620348,22.));
#15359=CARTESIAN_POINT('',(13.8083566691933,2.30852465794631,4.));
#15360=CARTESIAN_POINT('Origin',(0.,0.,4.));
#15361=CARTESIAN_POINT('',(13.8083566691933,2.30852465794631,1.));
#15362=CARTESIAN_POINT('',(13.8083566691933,2.30852465794631,22.));
#15363=CARTESIAN_POINT('Origin',(0.,0.,1.));
#15364=CARTESIAN_POINT('',(-13.8083566691933,2.30852465794631,4.));
#15365=CARTESIAN_POINT('',(-13.8083566691933,2.30852465794631,1.));
#15366=CARTESIAN_POINT('',(-13.8083566691933,2.30852465794631,22.));
#15367=CARTESIAN_POINT('',(-13.8459009408029,2.07147945620348,4.));
#15368=CARTESIAN_POINT('Origin',(0.,0.,4.));
#15369=CARTESIAN_POINT('',(-13.8459009408029,2.07147945620348,1.));
#15370=CARTESIAN_POINT('',(-13.8459009408029,2.07147945620348,22.));
#15371=CARTESIAN_POINT('Origin',(0.,0.,1.));
#15372=CARTESIAN_POINT('',(-13.2772200650433,4.4402057772599,4.));
#15373=CARTESIAN_POINT('',(-13.2772200650433,4.4402057772599,1.));
#15374=CARTESIAN_POINT('',(-13.2772200650433,4.4402057772599,22.));
#15375=CARTESIAN_POINT('',(-13.3513841436933,4.21195221334907,4.));
#15376=CARTESIAN_POINT('Origin',(0.,0.,4.));
#15377=CARTESIAN_POINT('',(-13.3513841436933,4.21195221334907,1.));
#15378=CARTESIAN_POINT('',(-13.3513841436933,4.21195221334907,22.));
#15379=CARTESIAN_POINT('Origin',(0.,0.,1.));
#15380=CARTESIAN_POINT('',(-12.4191542383249,6.46255429413924,4.));
#15381=CARTESIAN_POINT('',(-12.4191542383249,6.46255429413924,1.));
#15382=CARTESIAN_POINT('',(-12.4191542383249,6.46255429413924,22.));
#15383=CARTESIAN_POINT('',(-12.5281119582624,6.24871272833403,4.));
#15384=CARTESIAN_POINT('Origin',(0.,0.,4.));
#15385=CARTESIAN_POINT('',(-12.5281119582624,6.24871272833403,1.));
#15386=CARTESIAN_POINT('',(-12.5281119582624,6.24871272833403,22.));
#15387=CARTESIAN_POINT('Origin',(0.,0.,1.));
#15388=CARTESIAN_POINT('',(-11.255287617449,8.32577327630884,4.));
#15389=CARTESIAN_POINT('',(-11.255287617449,8.32577327630884,1.));
#15390=CARTESIAN_POINT('',(-11.255287617449,8.32577327630884,22.));
#15391=CARTESIAN_POINT('',(-11.3963560779992,8.13160919765885,4.));
#15392=CARTESIAN_POINT('Origin',(0.,0.,4.));
#15393=CARTESIAN_POINT('',(-11.3963560779992,8.13160919765885,1.));
#15394=CARTESIAN_POINT('',(-11.3963560779992,8.13160919765885,22.));
#15395=CARTESIAN_POINT('Origin',(0.,0.,1.));
#15396=CARTESIAN_POINT('',(-8.13160919765885,11.3963560779992,4.));
#15397=CARTESIAN_POINT('',(-8.13160919765885,11.3963560779992,1.));
#15398=CARTESIAN_POINT('',(-8.13160919765885,11.3963560779992,22.));
#15399=CARTESIAN_POINT('',(-8.32577327630884,11.255287617449,4.));
#15400=CARTESIAN_POINT('Origin',(0.,0.,4.));
#15401=CARTESIAN_POINT('',(-8.32577327630884,11.255287617449,1.));
#15402=CARTESIAN_POINT('',(-8.32577327630884,11.255287617449,22.));
#15403=CARTESIAN_POINT('Origin',(0.,0.,1.));
#15404=CARTESIAN_POINT('',(-6.24871272833403,12.5281119582624,4.));
#15405=CARTESIAN_POINT('',(-6.24871272833403,12.5281119582624,1.));
#15406=CARTESIAN_POINT('',(-6.24871272833403,12.5281119582624,22.));
#15407=CARTESIAN_POINT('',(-6.46255429413924,12.4191542383249,4.));
#15408=CARTESIAN_POINT('Origin',(0.,0.,4.));
#15409=CARTESIAN_POINT('',(-6.46255429413924,12.4191542383249,1.));
#15410=CARTESIAN_POINT('',(-6.46255429413924,12.4191542383249,22.));
#15411=CARTESIAN_POINT('Origin',(0.,0.,1.));
#15412=CARTESIAN_POINT('',(-4.21195221334906,13.3513841436933,4.));
#15413=CARTESIAN_POINT('',(-4.21195221334906,13.3513841436933,1.));
#15414=CARTESIAN_POINT('',(-4.21195221334906,13.3513841436933,22.));
#15415=CARTESIAN_POINT('',(-4.4402057772599,13.2772200650433,4.));
#15416=CARTESIAN_POINT('Origin',(0.,0.,4.));
#15417=CARTESIAN_POINT('',(-4.4402057772599,13.2772200650433,1.));
#15418=CARTESIAN_POINT('',(-4.4402057772599,13.2772200650433,22.));
#15419=CARTESIAN_POINT('Origin',(0.,0.,1.));
#15420=CARTESIAN_POINT('',(-2.07147945620348,13.8459009408029,4.));
#15421=CARTESIAN_POINT('',(-2.07147945620348,13.8459009408029,1.));
#15422=CARTESIAN_POINT('',(-2.07147945620348,13.8459009408029,22.));
#15423=CARTESIAN_POINT('',(-2.30852465794631,13.8083566691933,4.));
#15424=CARTESIAN_POINT('Origin',(0.,0.,4.));
#15425=CARTESIAN_POINT('',(-2.30852465794631,13.8083566691933,1.));
#15426=CARTESIAN_POINT('',(-2.30852465794631,13.8083566691933,22.));
#15427=CARTESIAN_POINT('Origin',(0.,0.,1.));
#15428=CARTESIAN_POINT('',(2.30852465794631,13.8083566691933,4.));
#15429=CARTESIAN_POINT('',(2.30852465794631,13.8083566691933,1.));
#15430=CARTESIAN_POINT('',(2.30852465794631,13.8083566691933,22.));
#15431=CARTESIAN_POINT('',(2.07147945620348,13.8459009408029,4.));
#15432=CARTESIAN_POINT('Origin',(0.,0.,4.));
#15433=CARTESIAN_POINT('',(2.07147945620348,13.8459009408029,1.));
#15434=CARTESIAN_POINT('',(2.07147945620348,13.8459009408029,22.));
#15435=CARTESIAN_POINT('Origin',(0.,0.,1.));
#15436=CARTESIAN_POINT('',(4.4402057772599,13.2772200650433,4.));
#15437=CARTESIAN_POINT('',(4.4402057772599,13.2772200650433,1.));
#15438=CARTESIAN_POINT('',(4.4402057772599,13.2772200650433,22.));
#15439=CARTESIAN_POINT('',(4.21195221334907,13.3513841436933,4.));
#15440=CARTESIAN_POINT('Origin',(0.,0.,4.));
#15441=CARTESIAN_POINT('',(4.21195221334907,13.3513841436933,1.));
#15442=CARTESIAN_POINT('',(4.21195221334907,13.3513841436933,22.));
#15443=CARTESIAN_POINT('Origin',(0.,0.,1.));
#15444=CARTESIAN_POINT('',(6.46255429413924,12.4191542383249,4.));
#15445=CARTESIAN_POINT('',(6.46255429413924,12.4191542383249,1.));
#15446=CARTESIAN_POINT('',(6.46255429413924,12.4191542383249,22.));
#15447=CARTESIAN_POINT('',(6.24871272833403,12.5281119582624,4.));
#15448=CARTESIAN_POINT('Origin',(0.,0.,4.));
#15449=CARTESIAN_POINT('',(6.24871272833403,12.5281119582624,1.));
#15450=CARTESIAN_POINT('',(6.24871272833403,12.5281119582624,22.));
#15451=CARTESIAN_POINT('Origin',(0.,0.,1.));
#15452=CARTESIAN_POINT('',(8.32577327630884,11.255287617449,4.));
#15453=CARTESIAN_POINT('',(8.32577327630884,11.255287617449,1.));
#15454=CARTESIAN_POINT('',(8.32577327630884,11.255287617449,22.));
#15455=CARTESIAN_POINT('',(8.13160919765885,11.3963560779992,4.));
#15456=CARTESIAN_POINT('Origin',(0.,0.,4.));
#15457=CARTESIAN_POINT('',(8.13160919765885,11.3963560779992,1.));
#15458=CARTESIAN_POINT('',(8.13160919765885,11.3963560779992,22.));
#15459=CARTESIAN_POINT('Origin',(0.,0.,1.));
#15460=CARTESIAN_POINT('',(11.3963560779992,8.13160919765885,4.));
#15461=CARTESIAN_POINT('',(11.3963560779992,8.13160919765885,1.));
#15462=CARTESIAN_POINT('',(11.3963560779992,8.13160919765885,22.));
#15463=CARTESIAN_POINT('',(11.255287617449,8.32577327630884,4.));
#15464=CARTESIAN_POINT('Origin',(0.,0.,4.));
#15465=CARTESIAN_POINT('',(11.255287617449,8.32577327630884,1.));
#15466=CARTESIAN_POINT('',(11.255287617449,8.32577327630884,22.));
#15467=CARTESIAN_POINT('Origin',(0.,0.,1.));
#15468=CARTESIAN_POINT('',(12.5281119582624,6.24871272833403,4.));
#15469=CARTESIAN_POINT('',(12.5281119582624,6.24871272833403,1.));
#15470=CARTESIAN_POINT('',(12.5281119582624,6.24871272833403,22.));
#15471=CARTESIAN_POINT('',(12.4191542383249,6.46255429413924,4.));
#15472=CARTESIAN_POINT('Origin',(0.,0.,4.));
#15473=CARTESIAN_POINT('',(12.4191542383249,6.46255429413924,1.));
#15474=CARTESIAN_POINT('',(12.4191542383249,6.46255429413924,22.));
#15475=CARTESIAN_POINT('Origin',(0.,0.,1.));
#15476=CARTESIAN_POINT('',(13.3513841436933,4.21195221334907,4.));
#15477=CARTESIAN_POINT('',(13.3513841436933,4.21195221334907,1.));
#15478=CARTESIAN_POINT('',(13.3513841436933,4.21195221334907,22.));
#15479=CARTESIAN_POINT('',(13.2772200650433,4.4402057772599,4.));
#15480=CARTESIAN_POINT('Origin',(0.,0.,4.));
#15481=CARTESIAN_POINT('',(13.2772200650433,4.4402057772599,1.));
#15482=CARTESIAN_POINT('',(13.2772200650433,4.4402057772599,22.));
#15483=CARTESIAN_POINT('Origin',(0.,0.,1.));
#15484=CARTESIAN_POINT('Origin',(0.,0.,22.));
#15485=CARTESIAN_POINT('Origin',(0.,0.,0.));
#15486=CARTESIAN_POINT('Origin',(9.461088732276,-9.63079435976078,7.));
#15487=CARTESIAN_POINT('',(9.461088732276,-9.63079435976078,1.));
#15488=CARTESIAN_POINT('',(9.461088732276,-9.63079435976078,1.));
#15489=CARTESIAN_POINT('',(9.461088732276,-9.63079435976078,7.));
#15490=CARTESIAN_POINT('',(9.461088732276,-9.63079435976078,7.));
#15491=CARTESIAN_POINT('',(9.461088732276,-9.63079435976078,7.));
#15492=CARTESIAN_POINT('Origin',(10.2671904628287,-10.0974848353439,7.));
#15493=CARTESIAN_POINT('',(9.63079435976077,-9.46108873227601,7.));
#15494=CARTESIAN_POINT('',(10.2671904628287,-10.0974848353439,7.));
#15495=CARTESIAN_POINT('',(9.63079435976077,-9.46108873227601,1.));
#15496=CARTESIAN_POINT('',(9.63079435976077,-9.46108873227601,7.));
#15497=CARTESIAN_POINT('',(10.2671904628287,-10.0974848353439,1.));
#15498=CARTESIAN_POINT('Origin',(0.,0.,7.));
#15499=CARTESIAN_POINT('',(9.63079435976077,-9.46108873227601,7.));
#15500=CARTESIAN_POINT('Origin',(0.,0.,1.));
#15501=CARTESIAN_POINT('',(9.63079435976077,-9.46108873227601,1.));
#15502=CARTESIAN_POINT('Origin',(9.63079435976077,-9.46108873227601,7.));
#15503=CARTESIAN_POINT('Origin',(-0.120000000000002,-13.5,7.));
#15504=CARTESIAN_POINT('',(-0.120000000000002,-13.5,1.));
#15505=CARTESIAN_POINT('',(-0.120000000000002,-13.5,1.));
#15506=CARTESIAN_POINT('',(-0.120000000000002,-13.5,7.));
#15507=CARTESIAN_POINT('',(-0.120000000000002,-13.5,7.));
#15508=CARTESIAN_POINT('',(-0.120000000000002,-13.5,7.));
#15509=CARTESIAN_POINT('Origin',(0.119999999999997,-14.4,7.));
#15510=CARTESIAN_POINT('',(0.119999999999998,-13.5,7.));
#15511=CARTESIAN_POINT('',(0.119999999999997,-14.4,7.));
#15512=CARTESIAN_POINT('',(0.119999999999998,-13.5,1.));
#15513=CARTESIAN_POINT('',(0.119999999999998,-13.5,7.));
#15514=CARTESIAN_POINT('',(0.119999999999997,-14.4,1.));
#15515=CARTESIAN_POINT('Origin',(0.,0.,7.));
#15516=CARTESIAN_POINT('',(0.119999999999998,-13.5,7.));
#15517=CARTESIAN_POINT('Origin',(0.,0.,1.));
#15518=CARTESIAN_POINT('',(0.119999999999998,-13.5,1.));
#15519=CARTESIAN_POINT('Origin',(0.119999999999998,-13.5,7.));
#15520=CARTESIAN_POINT('Origin',(-9.63079435976078,-9.46108873227601,7.));
#15521=CARTESIAN_POINT('',(-9.63079435976078,-9.46108873227601,1.));
#15522=CARTESIAN_POINT('',(-9.63079435976078,-9.46108873227601,1.));
#15523=CARTESIAN_POINT('',(-9.63079435976078,-9.46108873227601,7.));
#15524=CARTESIAN_POINT('',(-9.63079435976078,-9.46108873227601,7.));
#15525=CARTESIAN_POINT('',(-9.63079435976078,-9.46108873227601,7.));
#15526=CARTESIAN_POINT('Origin',(-10.0974848353439,-10.2671904628287,7.));
#15527=CARTESIAN_POINT('',(-9.46108873227601,-9.63079435976078,7.));
#15528=CARTESIAN_POINT('',(-10.0974848353439,-10.2671904628287,7.));
#15529=CARTESIAN_POINT('',(-9.46108873227601,-9.63079435976078,1.));
#15530=CARTESIAN_POINT('',(-9.46108873227601,-9.63079435976078,7.));
#15531=CARTESIAN_POINT('',(-10.0974848353439,-10.2671904628287,1.));
#15532=CARTESIAN_POINT('Origin',(0.,0.,7.));
#15533=CARTESIAN_POINT('',(-9.46108873227601,-9.63079435976078,7.));
#15534=CARTESIAN_POINT('Origin',(0.,0.,1.));
#15535=CARTESIAN_POINT('',(-9.46108873227601,-9.63079435976078,1.));
#15536=CARTESIAN_POINT('Origin',(-9.46108873227601,-9.63079435976078,7.));
#15537=CARTESIAN_POINT('Origin',(-13.5,0.120000000000002,7.));
#15538=CARTESIAN_POINT('',(-13.5,0.120000000000002,1.));
#15539=CARTESIAN_POINT('',(-13.5,0.120000000000002,1.));
#15540=CARTESIAN_POINT('',(-13.5,0.120000000000002,7.));
#15541=CARTESIAN_POINT('',(-13.5,0.120000000000002,7.));
#15542=CARTESIAN_POINT('',(-13.5,0.120000000000002,7.));
#15543=CARTESIAN_POINT('Origin',(-14.4,-0.119999999999998,7.));
#15544=CARTESIAN_POINT('',(-13.5,-0.119999999999998,7.));
#15545=CARTESIAN_POINT('',(-14.4,-0.119999999999998,7.));
#15546=CARTESIAN_POINT('',(-13.5,-0.119999999999998,1.));
#15547=CARTESIAN_POINT('',(-13.5,-0.119999999999998,7.));
#15548=CARTESIAN_POINT('',(-14.4,-0.119999999999998,1.));
#15549=CARTESIAN_POINT('Origin',(0.,0.,7.));
#15550=CARTESIAN_POINT('',(-13.5,-0.119999999999998,7.));
#15551=CARTESIAN_POINT('Origin',(0.,0.,1.));
#15552=CARTESIAN_POINT('',(-13.5,-0.119999999999998,1.));
#15553=CARTESIAN_POINT('Origin',(-13.5,-0.119999999999998,7.));
#15554=CARTESIAN_POINT('Origin',(-9.46108873227601,9.63079435976078,7.));
#15555=CARTESIAN_POINT('',(-9.46108873227601,9.63079435976078,1.));
#15556=CARTESIAN_POINT('',(-9.46108873227601,9.63079435976078,1.));
#15557=CARTESIAN_POINT('',(-9.46108873227601,9.63079435976078,7.));
#15558=CARTESIAN_POINT('',(-9.46108873227601,9.63079435976078,7.));
#15559=CARTESIAN_POINT('',(-9.46108873227601,9.63079435976078,7.));
#15560=CARTESIAN_POINT('Origin',(-10.2671904628287,10.0974848353439,7.));
#15561=CARTESIAN_POINT('',(-9.63079435976078,9.46108873227601,7.));
#15562=CARTESIAN_POINT('',(-10.2671904628287,10.0974848353439,7.));
#15563=CARTESIAN_POINT('',(-9.63079435976078,9.46108873227601,1.));
#15564=CARTESIAN_POINT('',(-9.63079435976078,9.46108873227601,7.));
#15565=CARTESIAN_POINT('',(-10.2671904628287,10.0974848353439,1.));
#15566=CARTESIAN_POINT('Origin',(0.,0.,7.));
#15567=CARTESIAN_POINT('',(-9.63079435976078,9.46108873227601,7.));
#15568=CARTESIAN_POINT('Origin',(0.,0.,1.));
#15569=CARTESIAN_POINT('',(-9.63079435976078,9.46108873227601,1.));
#15570=CARTESIAN_POINT('Origin',(-9.63079435976078,9.46108873227601,7.));
#15571=CARTESIAN_POINT('Origin',(0.120000000000001,13.5,7.));
#15572=CARTESIAN_POINT('',(0.120000000000001,13.5,1.));
#15573=CARTESIAN_POINT('',(0.120000000000001,13.5,1.));
#15574=CARTESIAN_POINT('',(0.120000000000001,13.5,7.));
#15575=CARTESIAN_POINT('',(0.120000000000001,13.5,7.));
#15576=CARTESIAN_POINT('',(0.120000000000001,13.5,7.));
#15577=CARTESIAN_POINT('Origin',(-0.119999999999999,14.4,7.));
#15578=CARTESIAN_POINT('',(-0.119999999999999,13.5,7.));
#15579=CARTESIAN_POINT('',(-0.119999999999999,14.4,7.));
#15580=CARTESIAN_POINT('',(-0.119999999999999,13.5,1.));
#15581=CARTESIAN_POINT('',(-0.119999999999999,13.5,7.));
#15582=CARTESIAN_POINT('',(-0.119999999999999,14.4,1.));
#15583=CARTESIAN_POINT('Origin',(0.,0.,7.));
#15584=CARTESIAN_POINT('',(-0.119999999999999,13.5,7.));
#15585=CARTESIAN_POINT('Origin',(0.,0.,1.));
#15586=CARTESIAN_POINT('',(-0.119999999999999,13.5,1.));
#15587=CARTESIAN_POINT('Origin',(-0.119999999999999,13.5,7.));
#15588=CARTESIAN_POINT('Origin',(9.63079435976078,9.46108873227601,7.));
#15589=CARTESIAN_POINT('',(9.63079435976078,9.46108873227601,1.));
#15590=CARTESIAN_POINT('',(9.63079435976078,9.46108873227601,1.));
#15591=CARTESIAN_POINT('',(9.63079435976078,9.46108873227601,7.));
#15592=CARTESIAN_POINT('',(9.63079435976078,9.46108873227601,7.));
#15593=CARTESIAN_POINT('',(9.63079435976078,9.46108873227601,7.));
#15594=CARTESIAN_POINT('Origin',(10.0974848353439,10.2671904628287,7.));
#15595=CARTESIAN_POINT('',(9.46108873227601,9.63079435976078,7.));
#15596=CARTESIAN_POINT('',(10.0974848353439,10.2671904628287,7.));
#15597=CARTESIAN_POINT('',(9.46108873227601,9.63079435976078,1.));
#15598=CARTESIAN_POINT('',(9.46108873227601,9.63079435976078,7.));
#15599=CARTESIAN_POINT('',(10.0974848353439,10.2671904628287,1.));
#15600=CARTESIAN_POINT('Origin',(0.,0.,7.));
#15601=CARTESIAN_POINT('',(9.46108873227601,9.63079435976078,7.));
#15602=CARTESIAN_POINT('Origin',(0.,0.,1.));
#15603=CARTESIAN_POINT('',(9.46108873227601,9.63079435976078,1.));
#15604=CARTESIAN_POINT('Origin',(9.46108873227601,9.63079435976078,7.));
#15605=CARTESIAN_POINT('Origin',(13.5,-0.12,7.));
#15606=CARTESIAN_POINT('',(13.5,-0.12,1.));
#15607=CARTESIAN_POINT('',(13.5,-0.12,1.));
#15608=CARTESIAN_POINT('',(13.5,-0.12,7.));
#15609=CARTESIAN_POINT('',(13.5,-0.12,7.));
#15610=CARTESIAN_POINT('',(13.5,-0.12,7.));
#15611=CARTESIAN_POINT('Origin',(14.4,0.12,7.));
#15612=CARTESIAN_POINT('',(13.5,0.12,7.));
#15613=CARTESIAN_POINT('',(14.4,0.12,7.));
#15614=CARTESIAN_POINT('',(13.5,0.12,1.));
#15615=CARTESIAN_POINT('',(13.5,0.12,7.));
#15616=CARTESIAN_POINT('',(14.4,0.12,1.));
#15617=CARTESIAN_POINT('Origin',(0.,0.,7.));
#15618=CARTESIAN_POINT('',(13.5,0.12,7.));
#15619=CARTESIAN_POINT('Origin',(0.,0.,1.));
#15620=CARTESIAN_POINT('',(13.5,0.12,1.));
#15621=CARTESIAN_POINT('Origin',(13.5,0.12,7.));
#15622=CARTESIAN_POINT('Origin',(13.3525647338392,1.9933426771717,4.));
#15623=CARTESIAN_POINT('',(13.3525647338392,1.9933426771717,1.));
#15624=CARTESIAN_POINT('',(13.3525647338392,1.9933426771717,1.));
#15625=CARTESIAN_POINT('',(13.3525647338392,1.9933426771717,4.));
#15626=CARTESIAN_POINT('',(13.3525647338392,1.9933426771717,4.));
#15627=CARTESIAN_POINT('',(13.3525647338392,1.9933426771717,4.));
#15628=CARTESIAN_POINT('Origin',(14.2039399687652,2.37117889745074,4.));
#15629=CARTESIAN_POINT('',(13.3150204622295,2.23038787891453,4.));
#15630=CARTESIAN_POINT('',(14.2039399687652,2.37117889745074,4.));
#15631=CARTESIAN_POINT('',(13.3150204622295,2.23038787891453,1.));
#15632=CARTESIAN_POINT('',(13.3150204622295,2.23038787891453,4.));
#15633=CARTESIAN_POINT('',(14.2039399687652,2.37117889745074,1.));
#15634=CARTESIAN_POINT('Origin',(0.,0.,4.));
#15635=CARTESIAN_POINT('',(13.3150204622295,2.23038787891453,4.));
#15636=CARTESIAN_POINT('Origin',(0.,0.,1.));
#15637=CARTESIAN_POINT('',(13.3150204622295,2.23038787891453,1.));
#15638=CARTESIAN_POINT('Origin',(13.3150204622295,2.23038787891453,4.));
#15639=CARTESIAN_POINT('Origin',(13.3150204622295,-2.23038787891454,4.));
#15640=CARTESIAN_POINT('',(13.3150204622295,-2.23038787891454,1.));
#15641=CARTESIAN_POINT('',(13.3150204622295,-2.23038787891454,1.));
#15642=CARTESIAN_POINT('',(13.3150204622295,-2.23038787891454,4.));
#15643=CARTESIAN_POINT('',(13.3150204622295,-2.23038787891454,4.));
#15644=CARTESIAN_POINT('',(13.3150204622295,-2.23038787891454,4.));
#15645=CARTESIAN_POINT('Origin',(14.2414842403748,-2.13413369570791,4.));
#15646=CARTESIAN_POINT('',(13.3525647338392,-1.9933426771717,4.));
#15647=CARTESIAN_POINT('',(14.2414842403748,-2.13413369570791,4.));
#15648=CARTESIAN_POINT('',(13.3525647338392,-1.9933426771717,1.));
#15649=CARTESIAN_POINT('',(13.3525647338392,-1.9933426771717,4.));
#15650=CARTESIAN_POINT('',(14.2414842403748,-2.13413369570791,1.));
#15651=CARTESIAN_POINT('Origin',(0.,0.,4.));
#15652=CARTESIAN_POINT('',(13.3525647338392,-1.9933426771717,4.));
#15653=CARTESIAN_POINT('Origin',(0.,0.,1.));
#15654=CARTESIAN_POINT('',(13.3525647338392,-1.9933426771717,1.));
#15655=CARTESIAN_POINT('Origin',(13.3525647338392,-1.9933426771717,4.));
#15656=CARTESIAN_POINT('Origin',(12.8021809306596,-4.28585620601721,4.));
#15657=CARTESIAN_POINT('',(12.8021809306596,-4.28585620601721,1.));
#15658=CARTESIAN_POINT('',(12.8021809306596,-4.28585620601721,1.));
#15659=CARTESIAN_POINT('',(12.8021809306596,-4.28585620601721,4.));
#15660=CARTESIAN_POINT('',(12.8021809306596,-4.28585620601721,4.));
#15661=CARTESIAN_POINT('',(12.8021809306596,-4.28585620601721,4.));
#15662=CARTESIAN_POINT('Origin',(13.7322958739752,-4.33571793704383,4.));
#15663=CARTESIAN_POINT('',(12.8763450093096,-4.05760264210638,4.));
#15664=CARTESIAN_POINT('',(13.7322958739752,-4.33571793704383,4.));
#15665=CARTESIAN_POINT('',(12.8763450093096,-4.05760264210638,1.));
#15666=CARTESIAN_POINT('',(12.8763450093096,-4.05760264210638,4.));
#15667=CARTESIAN_POINT('',(13.7322958739752,-4.33571793704383,1.));
#15668=CARTESIAN_POINT('Origin',(0.,0.,4.));
#15669=CARTESIAN_POINT('',(12.8763450093096,-4.05760264210638,4.));
#15670=CARTESIAN_POINT('Origin',(0.,0.,1.));
#15671=CARTESIAN_POINT('',(12.8763450093096,-4.05760264210638,1.));
#15672=CARTESIAN_POINT('Origin',(12.8763450093096,-4.05760264210638,4.));
#15673=CARTESIAN_POINT('Origin',(11.9741092165742,-6.23579252938649,4.));
#15674=CARTESIAN_POINT('',(11.9741092165742,-6.23579252938649,1.));
#15675=CARTESIAN_POINT('',(11.9741092165742,-6.23579252938649,1.));
#15676=CARTESIAN_POINT('',(11.9741092165742,-6.23579252938649,4.));
#15677=CARTESIAN_POINT('',(11.9741092165742,-6.23579252938649,4.));
#15678=CARTESIAN_POINT('',(11.9741092165742,-6.23579252938649,4.));
#15679=CARTESIAN_POINT('Origin',(12.8849728082812,-6.43054241334687,4.));
#15680=CARTESIAN_POINT('',(12.0830669365117,-6.02195096358128,4.));
#15681=CARTESIAN_POINT('',(12.8849728082812,-6.43054241334687,4.));
#15682=CARTESIAN_POINT('',(12.0830669365117,-6.02195096358128,1.));
#15683=CARTESIAN_POINT('',(12.0830669365117,-6.02195096358128,4.));
#15684=CARTESIAN_POINT('',(12.8849728082812,-6.43054241334687,1.));
#15685=CARTESIAN_POINT('Origin',(0.,0.,4.));
#15686=CARTESIAN_POINT('',(12.0830669365117,-6.02195096358128,4.));
#15687=CARTESIAN_POINT('Origin',(0.,0.,1.));
#15688=CARTESIAN_POINT('',(12.0830669365117,-6.02195096358128,1.));
#15689=CARTESIAN_POINT('Origin',(12.0830669365117,-6.02195096358128,4.));
#15690=CARTESIAN_POINT('Origin',(10.8511951937867,-8.03218294527338,4.));
#15691=CARTESIAN_POINT('',(10.8511951937867,-8.03218294527338,1.));
#15692=CARTESIAN_POINT('',(10.8511951937867,-8.03218294527338,1.));
#15693=CARTESIAN_POINT('',(10.8511951937867,-8.03218294527338,4.));
#15694=CARTESIAN_POINT('',(10.8511951937867,-8.03218294527338,4.));
#15695=CARTESIAN_POINT('',(10.8511951937867,-8.03218294527338,4.));
#15696=CARTESIAN_POINT('Origin',(11.7203789492743,-8.36702559368663,4.));
#15697=CARTESIAN_POINT('',(10.9922636543369,-7.8380188666234,4.));
#15698=CARTESIAN_POINT('',(11.7203789492743,-8.36702559368663,4.));
#15699=CARTESIAN_POINT('',(10.9922636543369,-7.8380188666234,1.));
#15700=CARTESIAN_POINT('',(10.9922636543369,-7.8380188666234,4.));
#15701=CARTESIAN_POINT('',(11.7203789492743,-8.36702559368663,1.));
#15702=CARTESIAN_POINT('Origin',(0.,0.,4.));
#15703=CARTESIAN_POINT('',(10.9922636543369,-7.8380188666234,4.));
#15704=CARTESIAN_POINT('Origin',(0.,0.,1.));
#15705=CARTESIAN_POINT('',(10.9922636543369,-7.8380188666234,1.));
#15706=CARTESIAN_POINT('Origin',(10.9922636543369,-7.8380188666234,4.));
#15707=CARTESIAN_POINT('Origin',(7.83801886662339,-10.9922636543369,4.));
#15708=CARTESIAN_POINT('',(7.83801886662339,-10.9922636543369,1.));
#15709=CARTESIAN_POINT('',(7.83801886662339,-10.9922636543369,1.));
#15710=CARTESIAN_POINT('',(7.83801886662339,-10.9922636543369,4.));
#15711=CARTESIAN_POINT('',(7.83801886662339,-10.9922636543369,4.));
#15712=CARTESIAN_POINT('',(7.83801886662339,-10.9922636543369,4.));
#15713=CARTESIAN_POINT('Origin',(8.5611896723366,-11.5793104887241,4.));
#15714=CARTESIAN_POINT('',(8.03218294527338,-10.8511951937867,4.));
#15715=CARTESIAN_POINT('',(8.5611896723366,-11.5793104887241,4.));
#15716=CARTESIAN_POINT('',(8.03218294527338,-10.8511951937867,1.));
#15717=CARTESIAN_POINT('',(8.03218294527338,-10.8511951937867,4.));
#15718=CARTESIAN_POINT('',(8.5611896723366,-11.5793104887241,1.));
#15719=CARTESIAN_POINT('Origin',(0.,0.,4.));
#15720=CARTESIAN_POINT('',(8.03218294527338,-10.8511951937867,4.));
#15721=CARTESIAN_POINT('Origin',(0.,0.,1.));
#15722=CARTESIAN_POINT('',(8.03218294527338,-10.8511951937867,1.));
#15723=CARTESIAN_POINT('Origin',(8.03218294527338,-10.8511951937867,4.));
#15724=CARTESIAN_POINT('Origin',(6.02195096358128,-12.0830669365117,4.));
#15725=CARTESIAN_POINT('',(6.02195096358128,-12.0830669365117,1.));
#15726=CARTESIAN_POINT('',(6.02195096358128,-12.0830669365117,1.));
#15727=CARTESIAN_POINT('',(6.02195096358128,-12.0830669365117,4.));
#15728=CARTESIAN_POINT('',(6.02195096358128,-12.0830669365117,4.));
#15729=CARTESIAN_POINT('',(6.02195096358128,-12.0830669365117,4.));
#15730=CARTESIAN_POINT('Origin',(6.64438397915208,-12.7760150883438,4.));
#15731=CARTESIAN_POINT('',(6.23579252938648,-11.9741092165742,4.));
#15732=CARTESIAN_POINT('',(6.64438397915208,-12.7760150883438,4.));
#15733=CARTESIAN_POINT('',(6.23579252938648,-11.9741092165742,1.));
#15734=CARTESIAN_POINT('',(6.23579252938648,-11.9741092165742,4.));
#15735=CARTESIAN_POINT('',(6.64438397915208,-12.7760150883438,1.));
#15736=CARTESIAN_POINT('Origin',(0.,0.,4.));
#15737=CARTESIAN_POINT('',(6.23579252938648,-11.9741092165742,4.));
#15738=CARTESIAN_POINT('Origin',(0.,0.,1.));
#15739=CARTESIAN_POINT('',(6.23579252938648,-11.9741092165742,1.));
#15740=CARTESIAN_POINT('Origin',(6.23579252938648,-11.9741092165742,4.));
#15741=CARTESIAN_POINT('Origin',(4.05760264210637,-12.8763450093096,4.));
#15742=CARTESIAN_POINT('',(4.05760264210637,-12.8763450093096,1.));
#15743=CARTESIAN_POINT('',(4.05760264210637,-12.8763450093096,1.));
#15744=CARTESIAN_POINT('',(4.05760264210637,-12.8763450093096,4.));
#15745=CARTESIAN_POINT('',(4.05760264210637,-12.8763450093096,4.));
#15746=CARTESIAN_POINT('',(4.05760264210637,-12.8763450093096,4.));
#15747=CARTESIAN_POINT('Origin',(4.56397150095466,-13.6581317953252,4.));
#15748=CARTESIAN_POINT('',(4.28585620601721,-12.8021809306596,4.));
#15749=CARTESIAN_POINT('',(4.56397150095466,-13.6581317953252,4.));
#15750=CARTESIAN_POINT('',(4.28585620601721,-12.8021809306596,1.));
#15751=CARTESIAN_POINT('',(4.28585620601721,-12.8021809306596,4.));
#15752=CARTESIAN_POINT('',(4.56397150095466,-13.6581317953252,1.));
#15753=CARTESIAN_POINT('Origin',(0.,0.,4.));
#15754=CARTESIAN_POINT('',(4.28585620601721,-12.8021809306596,4.));
#15755=CARTESIAN_POINT('Origin',(0.,0.,1.));
#15756=CARTESIAN_POINT('',(4.28585620601721,-12.8021809306596,1.));
#15757=CARTESIAN_POINT('Origin',(4.28585620601721,-12.8021809306596,4.));
#15758=CARTESIAN_POINT('Origin',(1.9933426771717,-13.3525647338392,4.));
#15759=CARTESIAN_POINT('',(1.9933426771717,-13.3525647338392,1.));
#15760=CARTESIAN_POINT('',(1.9933426771717,-13.3525647338392,1.));
#15761=CARTESIAN_POINT('',(1.9933426771717,-13.3525647338392,4.));
#15762=CARTESIAN_POINT('',(1.9933426771717,-13.3525647338392,4.));
#15763=CARTESIAN_POINT('',(1.9933426771717,-13.3525647338392,4.));
#15764=CARTESIAN_POINT('Origin',(2.37117889745074,-14.2039399687652,4.));
#15765=CARTESIAN_POINT('',(2.23038787891453,-13.3150204622295,4.));
#15766=CARTESIAN_POINT('',(2.37117889745074,-14.2039399687652,4.));
#15767=CARTESIAN_POINT('',(2.23038787891453,-13.3150204622295,1.));
#15768=CARTESIAN_POINT('',(2.23038787891453,-13.3150204622295,4.));
#15769=CARTESIAN_POINT('',(2.37117889745074,-14.2039399687652,1.));
#15770=CARTESIAN_POINT('Origin',(0.,0.,4.));
#15771=CARTESIAN_POINT('',(2.23038787891453,-13.3150204622295,4.));
#15772=CARTESIAN_POINT('Origin',(0.,0.,1.));
#15773=CARTESIAN_POINT('',(2.23038787891453,-13.3150204622295,1.));
#15774=CARTESIAN_POINT('Origin',(2.23038787891453,-13.3150204622295,4.));
#15775=CARTESIAN_POINT('Origin',(-2.23038787891454,-13.3150204622295,4.));
#15776=CARTESIAN_POINT('',(-2.23038787891454,-13.3150204622295,1.));
#15777=CARTESIAN_POINT('',(-2.23038787891454,-13.3150204622295,1.));
#15778=CARTESIAN_POINT('',(-2.23038787891454,-13.3150204622295,4.));
#15779=CARTESIAN_POINT('',(-2.23038787891454,-13.3150204622295,4.));
#15780=CARTESIAN_POINT('',(-2.23038787891454,-13.3150204622295,4.));
#15781=CARTESIAN_POINT('Origin',(-2.13413369570791,-14.2414842403748,4.));
#15782=CARTESIAN_POINT('',(-1.9933426771717,-13.3525647338392,4.));
#15783=CARTESIAN_POINT('',(-2.13413369570791,-14.2414842403748,4.));
#15784=CARTESIAN_POINT('',(-1.9933426771717,-13.3525647338392,1.));
#15785=CARTESIAN_POINT('',(-1.9933426771717,-13.3525647338392,4.));
#15786=CARTESIAN_POINT('',(-2.13413369570791,-14.2414842403748,1.));
#15787=CARTESIAN_POINT('Origin',(0.,0.,4.));
#15788=CARTESIAN_POINT('',(-1.9933426771717,-13.3525647338392,4.));
#15789=CARTESIAN_POINT('Origin',(0.,0.,1.));
#15790=CARTESIAN_POINT('',(-1.9933426771717,-13.3525647338392,1.));
#15791=CARTESIAN_POINT('Origin',(-1.9933426771717,-13.3525647338392,4.));
#15792=CARTESIAN_POINT('Origin',(-4.28585620601721,-12.8021809306596,4.));
#15793=CARTESIAN_POINT('',(-4.28585620601721,-12.8021809306596,1.));
#15794=CARTESIAN_POINT('',(-4.28585620601721,-12.8021809306596,1.));
#15795=CARTESIAN_POINT('',(-4.28585620601721,-12.8021809306596,4.));
#15796=CARTESIAN_POINT('',(-4.28585620601721,-12.8021809306596,4.));
#15797=CARTESIAN_POINT('',(-4.28585620601721,-12.8021809306596,4.));
#15798=CARTESIAN_POINT('Origin',(-4.33571793704383,-13.7322958739752,4.));
#15799=CARTESIAN_POINT('',(-4.05760264210637,-12.8763450093096,4.));
#15800=CARTESIAN_POINT('',(-4.33571793704383,-13.7322958739752,4.));
#15801=CARTESIAN_POINT('',(-4.05760264210637,-12.8763450093096,1.));
#15802=CARTESIAN_POINT('',(-4.05760264210637,-12.8763450093096,4.));
#15803=CARTESIAN_POINT('',(-4.33571793704383,-13.7322958739752,1.));
#15804=CARTESIAN_POINT('Origin',(0.,0.,4.));
#15805=CARTESIAN_POINT('',(-4.05760264210637,-12.8763450093096,4.));
#15806=CARTESIAN_POINT('Origin',(0.,0.,1.));
#15807=CARTESIAN_POINT('',(-4.05760264210637,-12.8763450093096,1.));
#15808=CARTESIAN_POINT('Origin',(-4.05760264210637,-12.8763450093096,4.));
#15809=CARTESIAN_POINT('Origin',(-6.23579252938649,-11.9741092165742,4.));
#15810=CARTESIAN_POINT('',(-6.23579252938649,-11.9741092165742,1.));
#15811=CARTESIAN_POINT('',(-6.23579252938649,-11.9741092165742,1.));
#15812=CARTESIAN_POINT('',(-6.23579252938649,-11.9741092165742,4.));
#15813=CARTESIAN_POINT('',(-6.23579252938649,-11.9741092165742,4.));
#15814=CARTESIAN_POINT('',(-6.23579252938649,-11.9741092165742,4.));
#15815=CARTESIAN_POINT('Origin',(-6.43054241334687,-12.8849728082812,4.));
#15816=CARTESIAN_POINT('',(-6.02195096358128,-12.0830669365117,4.));
#15817=CARTESIAN_POINT('',(-6.43054241334687,-12.8849728082812,4.));
#15818=CARTESIAN_POINT('',(-6.02195096358128,-12.0830669365117,1.));
#15819=CARTESIAN_POINT('',(-6.02195096358128,-12.0830669365117,4.));
#15820=CARTESIAN_POINT('',(-6.43054241334687,-12.8849728082812,1.));
#15821=CARTESIAN_POINT('Origin',(0.,0.,4.));
#15822=CARTESIAN_POINT('',(-6.02195096358128,-12.0830669365117,4.));
#15823=CARTESIAN_POINT('Origin',(0.,0.,1.));
#15824=CARTESIAN_POINT('',(-6.02195096358128,-12.0830669365117,1.));
#15825=CARTESIAN_POINT('Origin',(-6.02195096358128,-12.0830669365117,4.));
#15826=CARTESIAN_POINT('Origin',(-8.03218294527338,-10.8511951937867,4.));
#15827=CARTESIAN_POINT('',(-8.03218294527338,-10.8511951937867,1.));
#15828=CARTESIAN_POINT('',(-8.03218294527338,-10.8511951937867,1.));
#15829=CARTESIAN_POINT('',(-8.03218294527338,-10.8511951937867,4.));
#15830=CARTESIAN_POINT('',(-8.03218294527338,-10.8511951937867,4.));
#15831=CARTESIAN_POINT('',(-8.03218294527338,-10.8511951937867,4.));
#15832=CARTESIAN_POINT('Origin',(-8.36702559368662,-11.7203789492743,4.));
#15833=CARTESIAN_POINT('',(-7.8380188666234,-10.9922636543369,4.));
#15834=CARTESIAN_POINT('',(-8.36702559368662,-11.7203789492743,4.));
#15835=CARTESIAN_POINT('',(-7.8380188666234,-10.9922636543369,1.));
#15836=CARTESIAN_POINT('',(-7.8380188666234,-10.9922636543369,4.));
#15837=CARTESIAN_POINT('',(-8.36702559368662,-11.7203789492743,1.));
#15838=CARTESIAN_POINT('Origin',(0.,0.,4.));
#15839=CARTESIAN_POINT('',(-7.8380188666234,-10.9922636543369,4.));
#15840=CARTESIAN_POINT('Origin',(0.,0.,1.));
#15841=CARTESIAN_POINT('',(-7.8380188666234,-10.9922636543369,1.));
#15842=CARTESIAN_POINT('Origin',(-7.8380188666234,-10.9922636543369,4.));
#15843=CARTESIAN_POINT('Origin',(-10.9922636543369,-7.83801886662339,4.));
#15844=CARTESIAN_POINT('',(-10.9922636543369,-7.83801886662339,1.));
#15845=CARTESIAN_POINT('',(-10.9922636543369,-7.83801886662339,1.));
#15846=CARTESIAN_POINT('',(-10.9922636543369,-7.83801886662339,4.));
#15847=CARTESIAN_POINT('',(-10.9922636543369,-7.83801886662339,4.));
#15848=CARTESIAN_POINT('',(-10.9922636543369,-7.83801886662339,4.));
#15849=CARTESIAN_POINT('Origin',(-11.5793104887241,-8.5611896723366,4.));
#15850=CARTESIAN_POINT('',(-10.8511951937867,-8.03218294527338,4.));
#15851=CARTESIAN_POINT('',(-11.5793104887241,-8.5611896723366,4.));
#15852=CARTESIAN_POINT('',(-10.8511951937867,-8.03218294527338,1.));
#15853=CARTESIAN_POINT('',(-10.8511951937867,-8.03218294527338,4.));
#15854=CARTESIAN_POINT('',(-11.5793104887241,-8.5611896723366,1.));
#15855=CARTESIAN_POINT('Origin',(0.,0.,4.));
#15856=CARTESIAN_POINT('',(-10.8511951937867,-8.03218294527338,4.));
#15857=CARTESIAN_POINT('Origin',(0.,0.,1.));
#15858=CARTESIAN_POINT('',(-10.8511951937867,-8.03218294527338,1.));
#15859=CARTESIAN_POINT('Origin',(-10.8511951937867,-8.03218294527338,4.));
#15860=CARTESIAN_POINT('Origin',(-12.0830669365117,-6.02195096358128,4.));
#15861=CARTESIAN_POINT('',(-12.0830669365117,-6.02195096358128,1.));
#15862=CARTESIAN_POINT('',(-12.0830669365117,-6.02195096358128,1.));
#15863=CARTESIAN_POINT('',(-12.0830669365117,-6.02195096358128,4.));
#15864=CARTESIAN_POINT('',(-12.0830669365117,-6.02195096358128,4.));
#15865=CARTESIAN_POINT('',(-12.0830669365117,-6.02195096358128,4.));
#15866=CARTESIAN_POINT('Origin',(-12.7760150883438,-6.64438397915208,4.));
#15867=CARTESIAN_POINT('',(-11.9741092165742,-6.23579252938648,4.));
#15868=CARTESIAN_POINT('',(-12.7760150883438,-6.64438397915208,4.));
#15869=CARTESIAN_POINT('',(-11.9741092165742,-6.23579252938648,1.));
#15870=CARTESIAN_POINT('',(-11.9741092165742,-6.23579252938648,4.));
#15871=CARTESIAN_POINT('',(-12.7760150883438,-6.64438397915208,1.));
#15872=CARTESIAN_POINT('Origin',(0.,0.,4.));
#15873=CARTESIAN_POINT('',(-11.9741092165742,-6.23579252938648,4.));
#15874=CARTESIAN_POINT('Origin',(0.,0.,1.));
#15875=CARTESIAN_POINT('',(-11.9741092165742,-6.23579252938648,1.));
#15876=CARTESIAN_POINT('Origin',(-11.9741092165742,-6.23579252938648,4.));
#15877=CARTESIAN_POINT('Origin',(-12.8763450093096,-4.05760264210636,4.));
#15878=CARTESIAN_POINT('',(-12.8763450093096,-4.05760264210636,1.));
#15879=CARTESIAN_POINT('',(-12.8763450093096,-4.05760264210636,1.));
#15880=CARTESIAN_POINT('',(-12.8763450093096,-4.05760264210636,4.));
#15881=CARTESIAN_POINT('',(-12.8763450093096,-4.05760264210636,4.));
#15882=CARTESIAN_POINT('',(-12.8763450093096,-4.05760264210636,4.));
#15883=CARTESIAN_POINT('Origin',(-13.6581317953252,-4.56397150095465,4.));
#15884=CARTESIAN_POINT('',(-12.8021809306596,-4.2858562060172,4.));
#15885=CARTESIAN_POINT('',(-13.6581317953252,-4.56397150095465,4.));
#15886=CARTESIAN_POINT('',(-12.8021809306596,-4.2858562060172,1.));
#15887=CARTESIAN_POINT('',(-12.8021809306596,-4.2858562060172,4.));
#15888=CARTESIAN_POINT('',(-13.6581317953252,-4.56397150095465,1.));
#15889=CARTESIAN_POINT('Origin',(0.,0.,4.));
#15890=CARTESIAN_POINT('',(-12.8021809306596,-4.2858562060172,4.));
#15891=CARTESIAN_POINT('Origin',(0.,0.,1.));
#15892=CARTESIAN_POINT('',(-12.8021809306596,-4.2858562060172,1.));
#15893=CARTESIAN_POINT('Origin',(-12.8021809306596,-4.2858562060172,4.));
#15894=CARTESIAN_POINT('Origin',(-13.3525647338392,-1.9933426771717,4.));
#15895=CARTESIAN_POINT('',(-13.3525647338392,-1.9933426771717,1.));
#15896=CARTESIAN_POINT('',(-13.3525647338392,-1.9933426771717,1.));
#15897=CARTESIAN_POINT('',(-13.3525647338392,-1.9933426771717,4.));
#15898=CARTESIAN_POINT('',(-13.3525647338392,-1.9933426771717,4.));
#15899=CARTESIAN_POINT('',(-13.3525647338392,-1.9933426771717,4.));
#15900=CARTESIAN_POINT('Origin',(-14.2039399687652,-2.37117889745074,4.));
#15901=CARTESIAN_POINT('',(-13.3150204622295,-2.23038787891453,4.));
#15902=CARTESIAN_POINT('',(-14.2039399687652,-2.37117889745074,4.));
#15903=CARTESIAN_POINT('',(-13.3150204622295,-2.23038787891453,1.));
#15904=CARTESIAN_POINT('',(-13.3150204622295,-2.23038787891453,4.));
#15905=CARTESIAN_POINT('',(-14.2039399687652,-2.37117889745074,1.));
#15906=CARTESIAN_POINT('Origin',(0.,0.,4.));
#15907=CARTESIAN_POINT('',(-13.3150204622295,-2.23038787891453,4.));
#15908=CARTESIAN_POINT('Origin',(0.,0.,1.));
#15909=CARTESIAN_POINT('',(-13.3150204622295,-2.23038787891453,1.));
#15910=CARTESIAN_POINT('Origin',(-13.3150204622295,-2.23038787891453,4.));
#15911=CARTESIAN_POINT('Origin',(-13.3150204622295,2.23038787891453,4.));
#15912=CARTESIAN_POINT('',(-13.3150204622295,2.23038787891453,1.));
#15913=CARTESIAN_POINT('',(-13.3150204622295,2.23038787891453,1.));
#15914=CARTESIAN_POINT('',(-13.3150204622295,2.23038787891453,4.));
#15915=CARTESIAN_POINT('',(-13.3150204622295,2.23038787891453,4.));
#15916=CARTESIAN_POINT('',(-13.3150204622295,2.23038787891453,4.));
#15917=CARTESIAN_POINT('Origin',(-14.2414842403748,2.13413369570791,4.));
#15918=CARTESIAN_POINT('',(-13.3525647338392,1.9933426771717,4.));
#15919=CARTESIAN_POINT('',(-14.2414842403748,2.13413369570791,4.));
#15920=CARTESIAN_POINT('',(-13.3525647338392,1.9933426771717,1.));
#15921=CARTESIAN_POINT('',(-13.3525647338392,1.9933426771717,4.));
#15922=CARTESIAN_POINT('',(-14.2414842403748,2.13413369570791,1.));
#15923=CARTESIAN_POINT('Origin',(0.,0.,4.));
#15924=CARTESIAN_POINT('',(-13.3525647338392,1.9933426771717,4.));
#15925=CARTESIAN_POINT('Origin',(0.,0.,1.));
#15926=CARTESIAN_POINT('',(-13.3525647338392,1.9933426771717,1.));
#15927=CARTESIAN_POINT('Origin',(-13.3525647338392,1.9933426771717,4.));
#15928=CARTESIAN_POINT('Origin',(-12.8021809306596,4.28585620601721,4.));
#15929=CARTESIAN_POINT('',(-12.8021809306596,4.28585620601721,1.));
#15930=CARTESIAN_POINT('',(-12.8021809306596,4.28585620601721,1.));
#15931=CARTESIAN_POINT('',(-12.8021809306596,4.28585620601721,4.));
#15932=CARTESIAN_POINT('',(-12.8021809306596,4.28585620601721,4.));
#15933=CARTESIAN_POINT('',(-12.8021809306596,4.28585620601721,4.));
#15934=CARTESIAN_POINT('Origin',(-13.7322958739752,4.33571793704383,4.));
#15935=CARTESIAN_POINT('',(-12.8763450093096,4.05760264210637,4.));
#15936=CARTESIAN_POINT('',(-13.7322958739752,4.33571793704383,4.));
#15937=CARTESIAN_POINT('',(-12.8763450093096,4.05760264210637,1.));
#15938=CARTESIAN_POINT('',(-12.8763450093096,4.05760264210637,4.));
#15939=CARTESIAN_POINT('',(-13.7322958739752,4.33571793704383,1.));
#15940=CARTESIAN_POINT('Origin',(0.,0.,4.));
#15941=CARTESIAN_POINT('',(-12.8763450093096,4.05760264210637,4.));
#15942=CARTESIAN_POINT('Origin',(0.,0.,1.));
#15943=CARTESIAN_POINT('',(-12.8763450093096,4.05760264210637,1.));
#15944=CARTESIAN_POINT('Origin',(-12.8763450093096,4.05760264210637,4.));
#15945=CARTESIAN_POINT('Origin',(-11.9741092165742,6.23579252938649,4.));
#15946=CARTESIAN_POINT('',(-11.9741092165742,6.23579252938649,1.));
#15947=CARTESIAN_POINT('',(-11.9741092165742,6.23579252938649,1.));
#15948=CARTESIAN_POINT('',(-11.9741092165742,6.23579252938649,4.));
#15949=CARTESIAN_POINT('',(-11.9741092165742,6.23579252938649,4.));
#15950=CARTESIAN_POINT('',(-11.9741092165742,6.23579252938649,4.));
#15951=CARTESIAN_POINT('Origin',(-12.8849728082812,6.43054241334687,4.));
#15952=CARTESIAN_POINT('',(-12.0830669365117,6.02195096358128,4.));
#15953=CARTESIAN_POINT('',(-12.8849728082812,6.43054241334687,4.));
#15954=CARTESIAN_POINT('',(-12.0830669365117,6.02195096358128,1.));
#15955=CARTESIAN_POINT('',(-12.0830669365117,6.02195096358128,4.));
#15956=CARTESIAN_POINT('',(-12.8849728082812,6.43054241334687,1.));
#15957=CARTESIAN_POINT('Origin',(0.,0.,4.));
#15958=CARTESIAN_POINT('',(-12.0830669365117,6.02195096358128,4.));
#15959=CARTESIAN_POINT('Origin',(0.,0.,1.));
#15960=CARTESIAN_POINT('',(-12.0830669365117,6.02195096358128,1.));
#15961=CARTESIAN_POINT('Origin',(-12.0830669365117,6.02195096358128,4.));
#15962=CARTESIAN_POINT('Origin',(-10.8511951937867,8.03218294527338,4.));
#15963=CARTESIAN_POINT('',(-10.8511951937867,8.03218294527338,1.));
#15964=CARTESIAN_POINT('',(-10.8511951937867,8.03218294527338,1.));
#15965=CARTESIAN_POINT('',(-10.8511951937867,8.03218294527338,4.));
#15966=CARTESIAN_POINT('',(-10.8511951937867,8.03218294527338,4.));
#15967=CARTESIAN_POINT('',(-10.8511951937867,8.03218294527338,4.));
#15968=CARTESIAN_POINT('Origin',(-11.7203789492743,8.36702559368662,4.));
#15969=CARTESIAN_POINT('',(-10.9922636543369,7.8380188666234,4.));
#15970=CARTESIAN_POINT('',(-11.7203789492743,8.36702559368662,4.));
#15971=CARTESIAN_POINT('',(-10.9922636543369,7.8380188666234,1.));
#15972=CARTESIAN_POINT('',(-10.9922636543369,7.8380188666234,4.));
#15973=CARTESIAN_POINT('',(-11.7203789492743,8.36702559368662,1.));
#15974=CARTESIAN_POINT('Origin',(0.,0.,4.));
#15975=CARTESIAN_POINT('',(-10.9922636543369,7.8380188666234,4.));
#15976=CARTESIAN_POINT('Origin',(0.,0.,1.));
#15977=CARTESIAN_POINT('',(-10.9922636543369,7.8380188666234,1.));
#15978=CARTESIAN_POINT('Origin',(-10.9922636543369,7.8380188666234,4.));
#15979=CARTESIAN_POINT('Origin',(-7.83801886662339,10.9922636543369,4.));
#15980=CARTESIAN_POINT('',(-7.83801886662339,10.9922636543369,1.));
#15981=CARTESIAN_POINT('',(-7.83801886662339,10.9922636543369,1.));
#15982=CARTESIAN_POINT('',(-7.83801886662339,10.9922636543369,4.));
#15983=CARTESIAN_POINT('',(-7.83801886662339,10.9922636543369,4.));
#15984=CARTESIAN_POINT('',(-7.83801886662339,10.9922636543369,4.));
#15985=CARTESIAN_POINT('Origin',(-8.5611896723366,11.5793104887241,4.));
#15986=CARTESIAN_POINT('',(-8.03218294527338,10.8511951937867,4.));
#15987=CARTESIAN_POINT('',(-8.5611896723366,11.5793104887241,4.));
#15988=CARTESIAN_POINT('',(-8.03218294527338,10.8511951937867,1.));
#15989=CARTESIAN_POINT('',(-8.03218294527338,10.8511951937867,4.));
#15990=CARTESIAN_POINT('',(-8.5611896723366,11.5793104887241,1.));
#15991=CARTESIAN_POINT('Origin',(0.,0.,4.));
#15992=CARTESIAN_POINT('',(-8.03218294527338,10.8511951937867,4.));
#15993=CARTESIAN_POINT('Origin',(0.,0.,1.));
#15994=CARTESIAN_POINT('',(-8.03218294527338,10.8511951937867,1.));
#15995=CARTESIAN_POINT('Origin',(-8.03218294527338,10.8511951937867,4.));
#15996=CARTESIAN_POINT('Origin',(-6.02195096358128,12.0830669365117,4.));
#15997=CARTESIAN_POINT('',(-6.02195096358128,12.0830669365117,1.));
#15998=CARTESIAN_POINT('',(-6.02195096358128,12.0830669365117,1.));
#15999=CARTESIAN_POINT('',(-6.02195096358128,12.0830669365117,4.));
#16000=CARTESIAN_POINT('',(-6.02195096358128,12.0830669365117,4.));
#16001=CARTESIAN_POINT('',(-6.02195096358128,12.0830669365117,4.));
#16002=CARTESIAN_POINT('Origin',(-6.64438397915208,12.7760150883438,4.));
#16003=CARTESIAN_POINT('',(-6.23579252938649,11.9741092165742,4.));
#16004=CARTESIAN_POINT('',(-6.64438397915208,12.7760150883438,4.));
#16005=CARTESIAN_POINT('',(-6.23579252938649,11.9741092165742,1.));
#16006=CARTESIAN_POINT('',(-6.23579252938649,11.9741092165742,4.));
#16007=CARTESIAN_POINT('',(-6.64438397915208,12.7760150883438,1.));
#16008=CARTESIAN_POINT('Origin',(0.,0.,4.));
#16009=CARTESIAN_POINT('',(-6.23579252938649,11.9741092165742,4.));
#16010=CARTESIAN_POINT('Origin',(0.,0.,1.));
#16011=CARTESIAN_POINT('',(-6.23579252938649,11.9741092165742,1.));
#16012=CARTESIAN_POINT('Origin',(-6.23579252938649,11.9741092165742,4.));
#16013=CARTESIAN_POINT('Origin',(-4.05760264210637,12.8763450093096,4.));
#16014=CARTESIAN_POINT('',(-4.05760264210637,12.8763450093096,1.));
#16015=CARTESIAN_POINT('',(-4.05760264210637,12.8763450093096,1.));
#16016=CARTESIAN_POINT('',(-4.05760264210637,12.8763450093096,4.));
#16017=CARTESIAN_POINT('',(-4.05760264210637,12.8763450093096,4.));
#16018=CARTESIAN_POINT('',(-4.05760264210637,12.8763450093096,4.));
#16019=CARTESIAN_POINT('Origin',(-4.56397150095466,13.6581317953252,4.));
#16020=CARTESIAN_POINT('',(-4.28585620601721,12.8021809306596,4.));
#16021=CARTESIAN_POINT('',(-4.56397150095466,13.6581317953252,4.));
#16022=CARTESIAN_POINT('',(-4.28585620601721,12.8021809306596,1.));
#16023=CARTESIAN_POINT('',(-4.28585620601721,12.8021809306596,4.));
#16024=CARTESIAN_POINT('',(-4.56397150095466,13.6581317953252,1.));
#16025=CARTESIAN_POINT('Origin',(0.,0.,4.));
#16026=CARTESIAN_POINT('',(-4.28585620601721,12.8021809306596,4.));
#16027=CARTESIAN_POINT('Origin',(0.,0.,1.));
#16028=CARTESIAN_POINT('',(-4.28585620601721,12.8021809306596,1.));
#16029=CARTESIAN_POINT('Origin',(-4.28585620601721,12.8021809306596,4.));
#16030=CARTESIAN_POINT('Origin',(-1.9933426771717,13.3525647338392,4.));
#16031=CARTESIAN_POINT('',(-1.9933426771717,13.3525647338392,1.));
#16032=CARTESIAN_POINT('',(-1.9933426771717,13.3525647338392,1.));
#16033=CARTESIAN_POINT('',(-1.9933426771717,13.3525647338392,4.));
#16034=CARTESIAN_POINT('',(-1.9933426771717,13.3525647338392,4.));
#16035=CARTESIAN_POINT('',(-1.9933426771717,13.3525647338392,4.));
#16036=CARTESIAN_POINT('Origin',(-2.37117889745074,14.2039399687652,4.));
#16037=CARTESIAN_POINT('',(-2.23038787891453,13.3150204622295,4.));
#16038=CARTESIAN_POINT('',(-2.37117889745074,14.2039399687652,4.));
#16039=CARTESIAN_POINT('',(-2.23038787891453,13.3150204622295,1.));
#16040=CARTESIAN_POINT('',(-2.23038787891453,13.3150204622295,4.));
#16041=CARTESIAN_POINT('',(-2.37117889745074,14.2039399687652,1.));
#16042=CARTESIAN_POINT('Origin',(0.,0.,4.));
#16043=CARTESIAN_POINT('',(-2.23038787891453,13.3150204622295,4.));
#16044=CARTESIAN_POINT('Origin',(0.,0.,1.));
#16045=CARTESIAN_POINT('',(-2.23038787891453,13.3150204622295,1.));
#16046=CARTESIAN_POINT('Origin',(-2.23038787891453,13.3150204622295,4.));
#16047=CARTESIAN_POINT('Origin',(2.23038787891453,13.3150204622295,4.));
#16048=CARTESIAN_POINT('',(2.23038787891453,13.3150204622295,1.));
#16049=CARTESIAN_POINT('',(2.23038787891453,13.3150204622295,1.));
#16050=CARTESIAN_POINT('',(2.23038787891453,13.3150204622295,4.));
#16051=CARTESIAN_POINT('',(2.23038787891453,13.3150204622295,4.));
#16052=CARTESIAN_POINT('',(2.23038787891453,13.3150204622295,4.));
#16053=CARTESIAN_POINT('Origin',(2.13413369570791,14.2414842403748,4.));
#16054=CARTESIAN_POINT('',(1.9933426771717,13.3525647338392,4.));
#16055=CARTESIAN_POINT('',(2.13413369570791,14.2414842403748,4.));
#16056=CARTESIAN_POINT('',(1.9933426771717,13.3525647338392,1.));
#16057=CARTESIAN_POINT('',(1.9933426771717,13.3525647338392,4.));
#16058=CARTESIAN_POINT('',(2.13413369570791,14.2414842403748,1.));
#16059=CARTESIAN_POINT('Origin',(0.,0.,4.));
#16060=CARTESIAN_POINT('',(1.9933426771717,13.3525647338392,4.));
#16061=CARTESIAN_POINT('Origin',(0.,0.,1.));
#16062=CARTESIAN_POINT('',(1.9933426771717,13.3525647338392,1.));
#16063=CARTESIAN_POINT('Origin',(1.9933426771717,13.3525647338392,4.));
#16064=CARTESIAN_POINT('Origin',(4.28585620601721,12.8021809306596,4.));
#16065=CARTESIAN_POINT('',(4.28585620601721,12.8021809306596,1.));
#16066=CARTESIAN_POINT('',(4.28585620601721,12.8021809306596,1.));
#16067=CARTESIAN_POINT('',(4.28585620601721,12.8021809306596,4.));
#16068=CARTESIAN_POINT('',(4.28585620601721,12.8021809306596,4.));
#16069=CARTESIAN_POINT('',(4.28585620601721,12.8021809306596,4.));
#16070=CARTESIAN_POINT('Origin',(4.33571793704383,13.7322958739752,4.));
#16071=CARTESIAN_POINT('',(4.05760264210637,12.8763450093096,4.));
#16072=CARTESIAN_POINT('',(4.33571793704383,13.7322958739752,4.));
#16073=CARTESIAN_POINT('',(4.05760264210637,12.8763450093096,1.));
#16074=CARTESIAN_POINT('',(4.05760264210637,12.8763450093096,4.));
#16075=CARTESIAN_POINT('',(4.33571793704383,13.7322958739752,1.));
#16076=CARTESIAN_POINT('Origin',(0.,0.,4.));
#16077=CARTESIAN_POINT('',(4.05760264210637,12.8763450093096,4.));
#16078=CARTESIAN_POINT('Origin',(0.,0.,1.));
#16079=CARTESIAN_POINT('',(4.05760264210637,12.8763450093096,1.));
#16080=CARTESIAN_POINT('Origin',(4.05760264210637,12.8763450093096,4.));
#16081=CARTESIAN_POINT('Origin',(6.23579252938649,11.9741092165742,4.));
#16082=CARTESIAN_POINT('',(6.23579252938649,11.9741092165742,1.));
#16083=CARTESIAN_POINT('',(6.23579252938649,11.9741092165742,1.));
#16084=CARTESIAN_POINT('',(6.23579252938649,11.9741092165742,4.));
#16085=CARTESIAN_POINT('',(6.23579252938649,11.9741092165742,4.));
#16086=CARTESIAN_POINT('',(6.23579252938649,11.9741092165742,4.));
#16087=CARTESIAN_POINT('Origin',(6.43054241334687,12.8849728082812,4.));
#16088=CARTESIAN_POINT('',(6.02195096358128,12.0830669365117,4.));
#16089=CARTESIAN_POINT('',(6.43054241334687,12.8849728082812,4.));
#16090=CARTESIAN_POINT('',(6.02195096358128,12.0830669365117,1.));
#16091=CARTESIAN_POINT('',(6.02195096358128,12.0830669365117,4.));
#16092=CARTESIAN_POINT('',(6.43054241334687,12.8849728082812,1.));
#16093=CARTESIAN_POINT('Origin',(0.,0.,4.));
#16094=CARTESIAN_POINT('',(6.02195096358128,12.0830669365117,4.));
#16095=CARTESIAN_POINT('Origin',(0.,0.,1.));
#16096=CARTESIAN_POINT('',(6.02195096358128,12.0830669365117,1.));
#16097=CARTESIAN_POINT('Origin',(6.02195096358128,12.0830669365117,4.));
#16098=CARTESIAN_POINT('Origin',(8.03218294527338,10.8511951937867,4.));
#16099=CARTESIAN_POINT('',(8.03218294527338,10.8511951937867,1.));
#16100=CARTESIAN_POINT('',(8.03218294527338,10.8511951937867,1.));
#16101=CARTESIAN_POINT('',(8.03218294527338,10.8511951937867,4.));
#16102=CARTESIAN_POINT('',(8.03218294527338,10.8511951937867,4.));
#16103=CARTESIAN_POINT('',(8.03218294527338,10.8511951937867,4.));
#16104=CARTESIAN_POINT('Origin',(8.36702559368662,11.7203789492743,4.));
#16105=CARTESIAN_POINT('',(7.8380188666234,10.9922636543369,4.));
#16106=CARTESIAN_POINT('',(8.36702559368662,11.7203789492743,4.));
#16107=CARTESIAN_POINT('',(7.8380188666234,10.9922636543369,1.));
#16108=CARTESIAN_POINT('',(7.8380188666234,10.9922636543369,4.));
#16109=CARTESIAN_POINT('',(8.36702559368662,11.7203789492743,1.));
#16110=CARTESIAN_POINT('Origin',(0.,0.,4.));
#16111=CARTESIAN_POINT('',(7.8380188666234,10.9922636543369,4.));
#16112=CARTESIAN_POINT('Origin',(0.,0.,1.));
#16113=CARTESIAN_POINT('',(7.8380188666234,10.9922636543369,1.));
#16114=CARTESIAN_POINT('Origin',(7.8380188666234,10.9922636543369,4.));
#16115=CARTESIAN_POINT('Origin',(10.9922636543369,7.8380188666234,4.));
#16116=CARTESIAN_POINT('',(10.9922636543369,7.8380188666234,1.));
#16117=CARTESIAN_POINT('',(10.9922636543369,7.8380188666234,1.));
#16118=CARTESIAN_POINT('',(10.9922636543369,7.8380188666234,4.));
#16119=CARTESIAN_POINT('',(10.9922636543369,7.8380188666234,4.));
#16120=CARTESIAN_POINT('',(10.9922636543369,7.8380188666234,4.));
#16121=CARTESIAN_POINT('Origin',(11.5793104887241,8.56118967233661,4.));
#16122=CARTESIAN_POINT('',(10.8511951937867,8.03218294527338,4.));
#16123=CARTESIAN_POINT('',(11.5793104887241,8.56118967233661,4.));
#16124=CARTESIAN_POINT('',(10.8511951937867,8.03218294527338,1.));
#16125=CARTESIAN_POINT('',(10.8511951937867,8.03218294527338,4.));
#16126=CARTESIAN_POINT('',(11.5793104887241,8.56118967233661,1.));
#16127=CARTESIAN_POINT('Origin',(0.,0.,4.));
#16128=CARTESIAN_POINT('',(10.8511951937867,8.03218294527338,4.));
#16129=CARTESIAN_POINT('Origin',(0.,0.,1.));
#16130=CARTESIAN_POINT('',(10.8511951937867,8.03218294527338,1.));
#16131=CARTESIAN_POINT('Origin',(10.8511951937867,8.03218294527338,4.));
#16132=CARTESIAN_POINT('Origin',(12.0830669365117,6.02195096358128,4.));
#16133=CARTESIAN_POINT('',(12.0830669365117,6.02195096358128,1.));
#16134=CARTESIAN_POINT('',(12.0830669365117,6.02195096358128,1.));
#16135=CARTESIAN_POINT('',(12.0830669365117,6.02195096358128,4.));
#16136=CARTESIAN_POINT('',(12.0830669365117,6.02195096358128,4.));
#16137=CARTESIAN_POINT('',(12.0830669365117,6.02195096358128,4.));
#16138=CARTESIAN_POINT('Origin',(12.7760150883438,6.64438397915208,4.));
#16139=CARTESIAN_POINT('',(11.9741092165742,6.23579252938649,4.));
#16140=CARTESIAN_POINT('',(12.7760150883438,6.64438397915208,4.));
#16141=CARTESIAN_POINT('',(11.9741092165742,6.23579252938649,1.));
#16142=CARTESIAN_POINT('',(11.9741092165742,6.23579252938649,4.));
#16143=CARTESIAN_POINT('',(12.7760150883438,6.64438397915208,1.));
#16144=CARTESIAN_POINT('Origin',(0.,0.,4.));
#16145=CARTESIAN_POINT('',(11.9741092165742,6.23579252938649,4.));
#16146=CARTESIAN_POINT('Origin',(0.,0.,1.));
#16147=CARTESIAN_POINT('',(11.9741092165742,6.23579252938649,1.));
#16148=CARTESIAN_POINT('Origin',(11.9741092165742,6.23579252938649,4.));
#16149=CARTESIAN_POINT('Origin',(12.8763450093096,4.05760264210637,4.));
#16150=CARTESIAN_POINT('',(12.8763450093096,4.05760264210637,1.));
#16151=CARTESIAN_POINT('',(12.8763450093096,4.05760264210637,1.));
#16152=CARTESIAN_POINT('',(12.8763450093096,4.05760264210637,4.));
#16153=CARTESIAN_POINT('',(12.8763450093096,4.05760264210637,4.));
#16154=CARTESIAN_POINT('',(12.8763450093096,4.05760264210637,4.));
#16155=CARTESIAN_POINT('Origin',(13.6581317953252,4.56397150095466,4.));
#16156=CARTESIAN_POINT('',(12.8021809306596,4.28585620601721,4.));
#16157=CARTESIAN_POINT('',(13.6581317953252,4.56397150095466,4.));
#16158=CARTESIAN_POINT('',(12.8021809306596,4.28585620601721,1.));
#16159=CARTESIAN_POINT('',(12.8021809306596,4.28585620601721,4.));
#16160=CARTESIAN_POINT('',(13.6581317953252,4.56397150095466,1.));
#16161=CARTESIAN_POINT('Origin',(0.,0.,4.));
#16162=CARTESIAN_POINT('',(12.8021809306596,4.28585620601721,4.));
#16163=CARTESIAN_POINT('Origin',(0.,0.,1.));
#16164=CARTESIAN_POINT('',(12.8021809306596,4.28585620601721,1.));
#16165=CARTESIAN_POINT('Origin',(12.8021809306596,4.28585620601721,4.));
#16564=UNCERTAINTY_MEASURE_WITH_UNIT(LENGTH_MEASURE(0.01),#16599,
'DISTANCE_ACCURACY_VALUE',
'Maximum model space distance between geometric entities at asserted c
onnectivities');
#16572=UNCERTAINTY_MEASURE_WITH_UNIT(LENGTH_MEASURE(0.01),#16599,
'DISTANCE_ACCURACY_VALUE',
'Maximum model space distance between geometric entities at asserted c
onnectivities');
#16590=(
GEOMETRIC_REPRESENTATION_CONTEXT(3)
GLOBAL_UNCERTAINTY_ASSIGNED_CONTEXT((#16564))
GLOBAL_UNIT_ASSIGNED_CONTEXT((#16599,#16601,#16602))
REPRESENTATION_CONTEXT('','3D')
);
#16598=(
GEOMETRIC_REPRESENTATION_CONTEXT(3)
GLOBAL_UNCERTAINTY_ASSIGNED_CONTEXT((#16572))
GLOBAL_UNIT_ASSIGNED_CONTEXT((#16599,#16601,#16602))
REPRESENTATION_CONTEXT('','3D')
);
#16599=(
LENGTH_UNIT()
NAMED_UNIT(*)
SI_UNIT(.MILLI.,.METRE.)
);
#16601=(
NAMED_UNIT(*)
PLANE_ANGLE_UNIT()
SI_UNIT($,.RADIAN.)
);
#16602=(
NAMED_UNIT(*)
SI_UNIT($,.STERADIAN.)
SOLID_ANGLE_UNIT()
);
#16620=SHAPE_DEFINITION_REPRESENTATION(#16645,#16714);
#16645=PRODUCT_DEFINITION_SHAPE('',$,#16740);
#16714=SHAPE_REPRESENTATION('',(#10487),#16590);
#16722=PRODUCT_DEFINITION_CONTEXT('part definition',#16799,'design');
#16740=PRODUCT_DEFINITION('P15_Graduated_Feed_Dial',
'P15_Graduated_Feed_Dial',#16765,#16722);
#16765=PRODUCT_DEFINITION_FORMATION('',$,#16818);
#16799=APPLICATION_CONTEXT(
'Core Data for Automotive Mechanical Design Process');
#16800=PRODUCT_CONTEXT('part definition',#16799,'mechanical');
#16818=PRODUCT('P15_Graduated_Feed_Dial','P15_Graduated_Feed_Dial',$,(#16800));
#16834=PRESENTATION_STYLE_ASSIGNMENT((#16843));
#16843=SURFACE_STYLE_USAGE(.BOTH.,#16852);
#16852=SURFACE_SIDE_STYLE('',(#16861));
#16861=SURFACE_STYLE_FILL_AREA(#16870);
#16870=FILL_AREA_STYLE('Light Blue',(#16879));
#16879=FILL_AREA_STYLE_COLOUR('Light Blue',#16888);
#16888=COLOUR_RGB('Light Blue',0.67843137254902,0.847058823529412,0.901960784313726);
ENDSEC;
END-ISO-10303-21;
